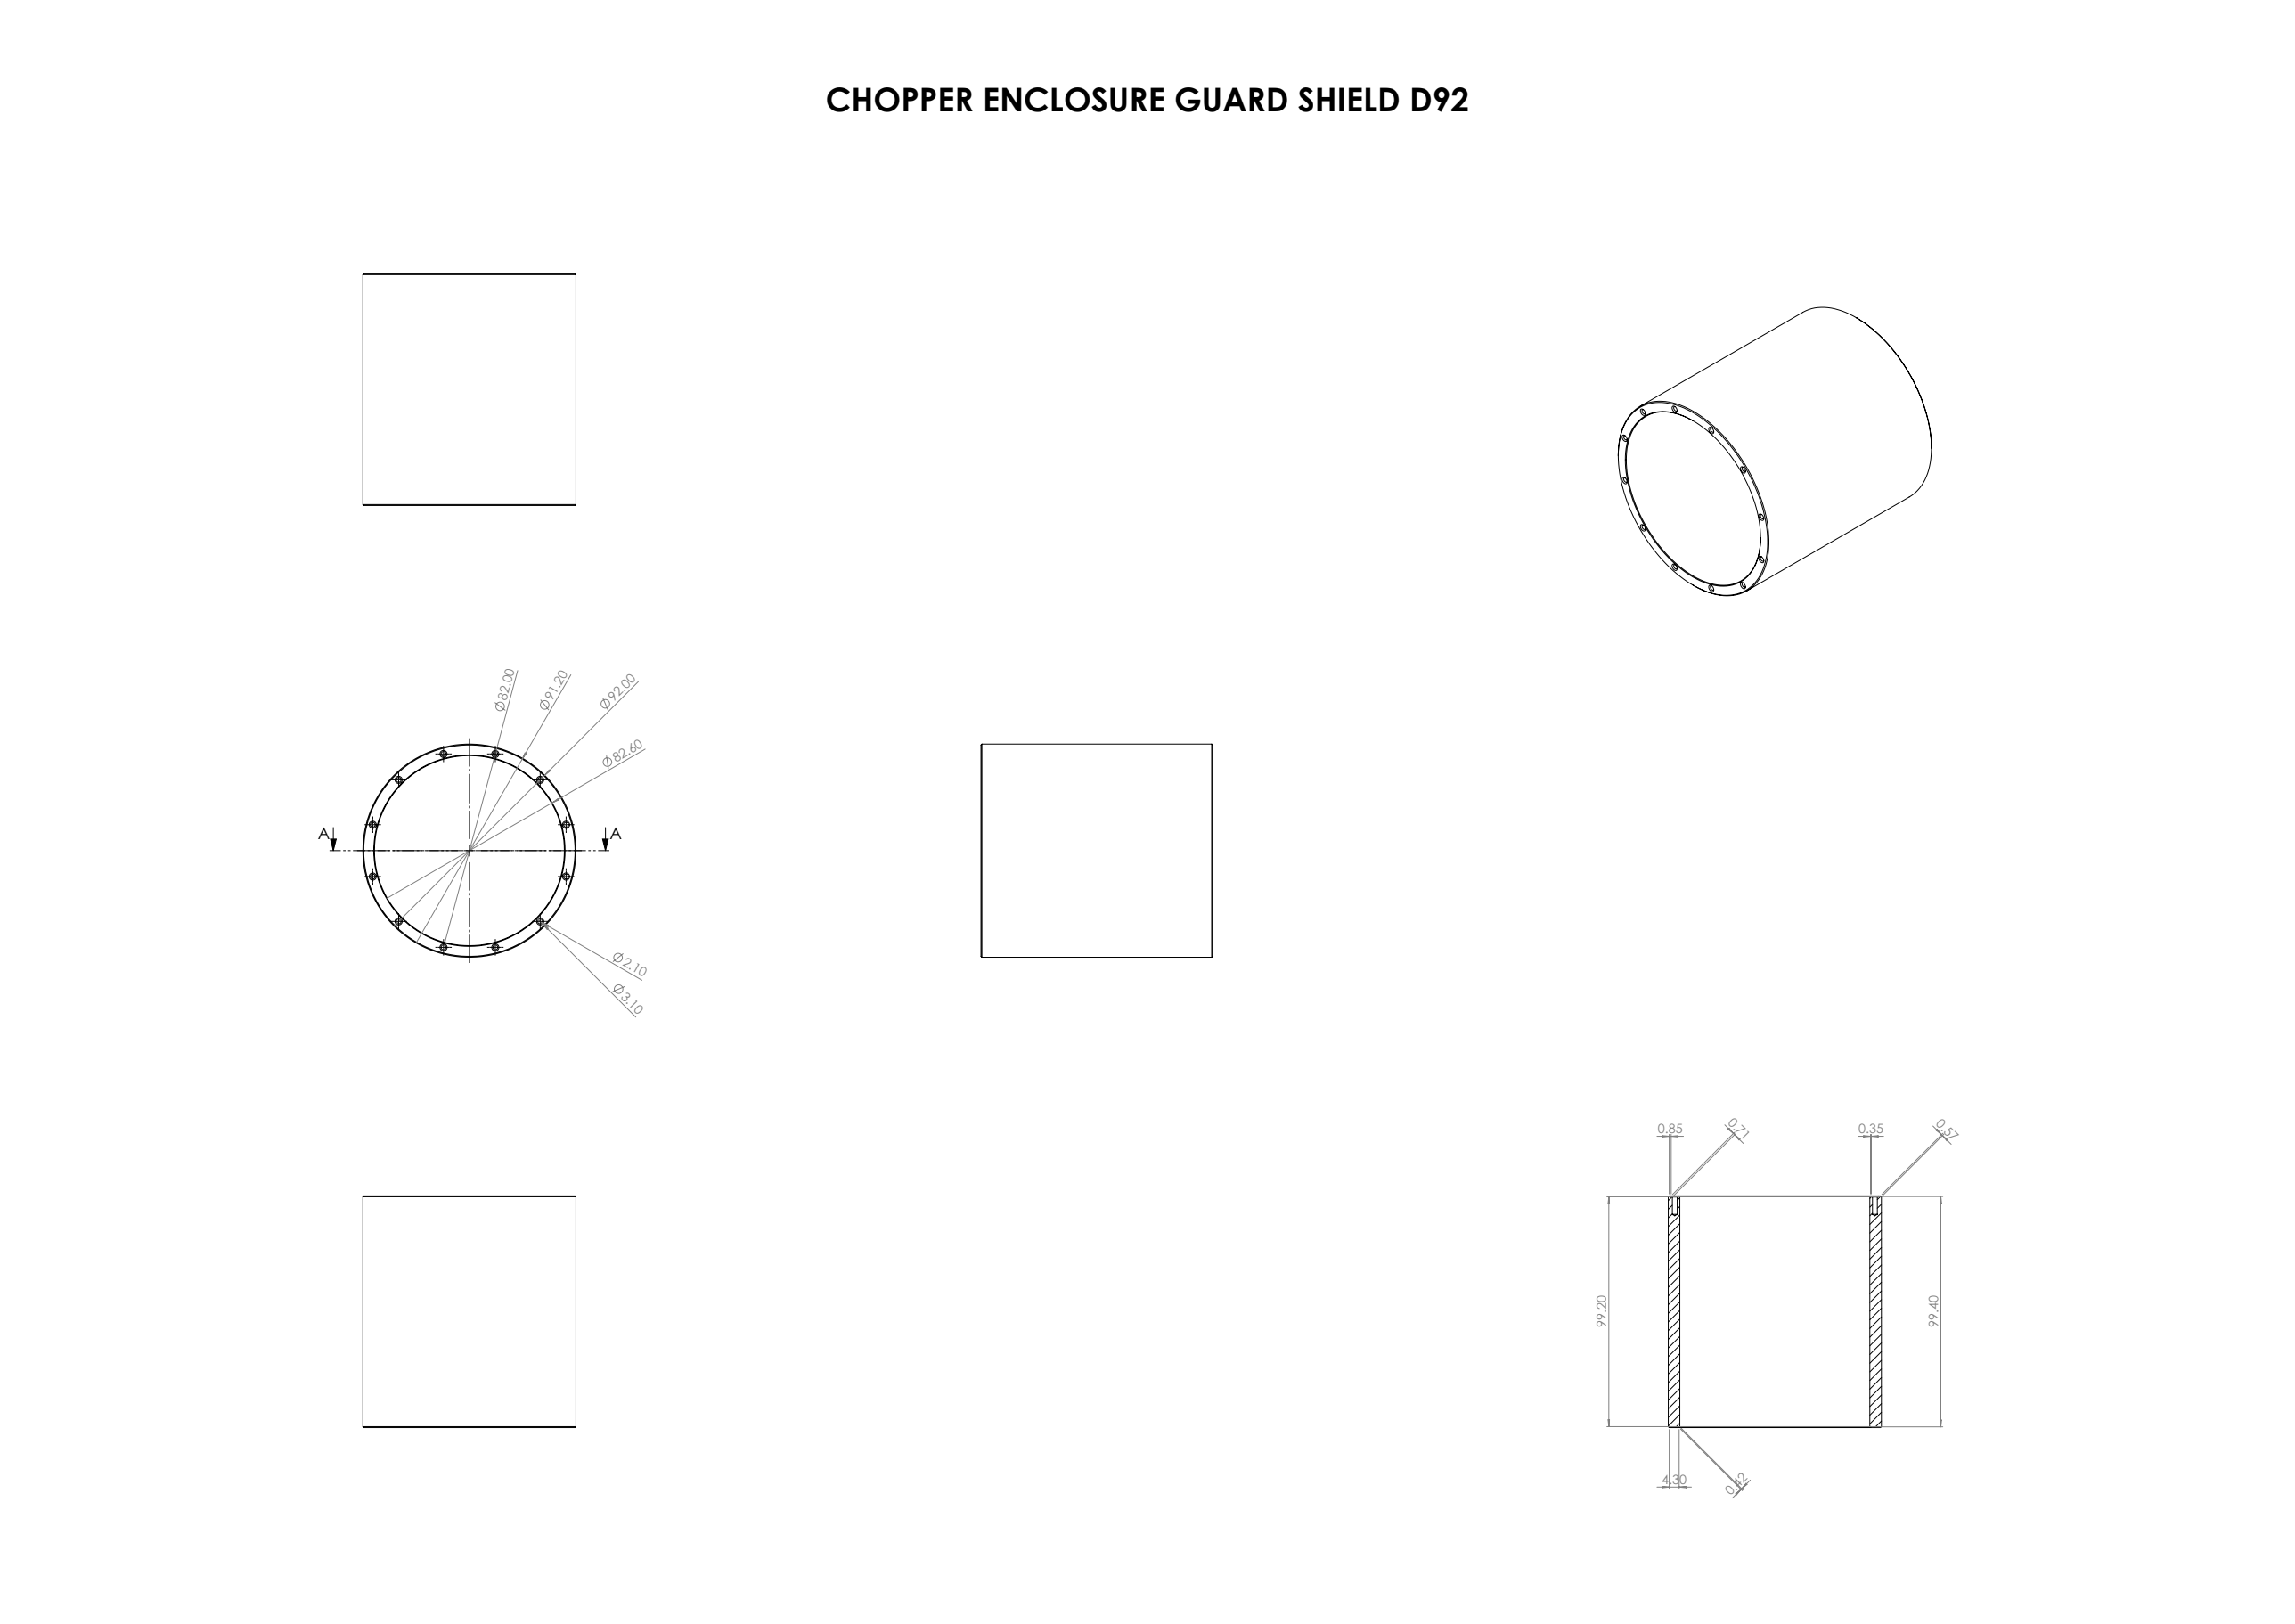
ISO-10303-21;
HEADER;
/* Generated by software containing ST-Developer
 * from STEP Tools, Inc. (www.steptools.com) 
 */

FILE_DESCRIPTION(
/* description */ (''),
/* implementation_level */ '2;1');

FILE_NAME(
/* name */ '02_Chopper_Enclosure_Guard_Shield_D92.step',
/* time_stamp */ '2026-10-19T23:00:43-07:00',
/* author */ (''),
/* organization */ (''),
/* preprocessor_version */ 'ST-DEVELOPER v20.2',
/* originating_system */ 'Autodesk Translation Framework v15.15.0.0',
/* authorisation */ '');

FILE_SCHEMA (('AUTOMOTIVE_DESIGN { 1 0 10303 214 3 1 1 }'));
ENDSEC;

DATA;
#10=MECHANICAL_DESIGN_GEOMETRIC_PRESENTATION_REPRESENTATION('',(#997),#55002);
#957=SHAPE_REPRESENTATION_RELATIONSHIP('SRR','None',#55105,#977);
#977=ADVANCED_BREP_SHAPE_REPRESENTATION('',(#1017),#54983);
#997=STYLED_ITEM('',(#55379),#1017);
#1017=MANIFOLD_SOLID_BREP('Enclosure Guard Shield',#24530);
#1062=FACE_BOUND('',#3929,.T.);
#1063=FACE_BOUND('',#3930,.T.);
#1064=FACE_BOUND('',#3931,.T.);
#1065=FACE_BOUND('',#3932,.T.);
#1066=FACE_BOUND('',#3933,.T.);
#1067=FACE_BOUND('',#3934,.T.);
#1068=FACE_BOUND('',#3935,.T.);
#1069=FACE_BOUND('',#3938,.T.);
#1070=FACE_BOUND('',#3939,.T.);
#1071=FACE_BOUND('',#3940,.T.);
#1072=FACE_BOUND('',#3941,.T.);
#1073=FACE_BOUND('',#3942,.T.);
#1074=FACE_BOUND('',#3943,.T.);
#1075=FACE_BOUND('',#3944,.T.);
#1076=FACE_BOUND('',#3945,.T.);
#1077=FACE_BOUND('',#3946,.T.);
#1078=FACE_BOUND('',#3947,.T.);
#1079=FACE_BOUND('',#3948,.T.);
#1080=FACE_BOUND('',#3949,.T.);
#1081=FACE_BOUND('',#3950,.T.);
#1287=PLANE('',#25045);
#1288=PLANE('',#25049);
#1972=CYLINDRICAL_SURFACE('',#24932,0.105);
#1973=CYLINDRICAL_SURFACE('',#24938,0.105);
#1974=CYLINDRICAL_SURFACE('',#24944,0.105);
#1975=CYLINDRICAL_SURFACE('',#24950,0.105);
#1976=CYLINDRICAL_SURFACE('',#24956,0.105);
#1977=CYLINDRICAL_SURFACE('',#24962,0.105);
#1978=CYLINDRICAL_SURFACE('',#24968,0.105);
#1979=CYLINDRICAL_SURFACE('',#24974,0.105);
#1980=CYLINDRICAL_SURFACE('',#24980,0.105);
#1981=CYLINDRICAL_SURFACE('',#24986,0.105);
#1982=CYLINDRICAL_SURFACE('',#24992,0.105);
#1983=CYLINDRICAL_SURFACE('',#24998,0.105);
#1984=CYLINDRICAL_SURFACE('',#25004,0.105);
#1985=CYLINDRICAL_SURFACE('',#25010,0.105);
#1986=CYLINDRICAL_SURFACE('',#25016,0.105);
#1987=CYLINDRICAL_SURFACE('',#25022,0.105);
#1988=CYLINDRICAL_SURFACE('',#25028,0.105);
#1989=CYLINDRICAL_SURFACE('',#25034,0.105);
#1990=CYLINDRICAL_SURFACE('',#25042,4.1);
#1991=CYLINDRICAL_SURFACE('',#25054,4.6);
#2482=FACE_OUTER_BOUND('',#3872,.T.);
#2483=FACE_OUTER_BOUND('',#3873,.T.);
#2484=FACE_OUTER_BOUND('',#3874,.T.);
#2485=FACE_OUTER_BOUND('',#3875,.T.);
#2486=FACE_OUTER_BOUND('',#3876,.T.);
#2487=FACE_OUTER_BOUND('',#3877,.T.);
#2488=FACE_OUTER_BOUND('',#3878,.T.);
#2489=FACE_OUTER_BOUND('',#3879,.T.);
#2490=FACE_OUTER_BOUND('',#3880,.T.);
#2491=FACE_OUTER_BOUND('',#3881,.T.);
#2492=FACE_OUTER_BOUND('',#3882,.T.);
#2493=FACE_OUTER_BOUND('',#3883,.T.);
#2494=FACE_OUTER_BOUND('',#3884,.T.);
#2495=FACE_OUTER_BOUND('',#3885,.T.);
#2496=FACE_OUTER_BOUND('',#3886,.T.);
#2497=FACE_OUTER_BOUND('',#3887,.T.);
#2498=FACE_OUTER_BOUND('',#3888,.T.);
#2499=FACE_OUTER_BOUND('',#3889,.T.);
#2500=FACE_OUTER_BOUND('',#3890,.T.);
#2501=FACE_OUTER_BOUND('',#3891,.T.);
#2502=FACE_OUTER_BOUND('',#3892,.T.);
#2503=FACE_OUTER_BOUND('',#3893,.T.);
#2504=FACE_OUTER_BOUND('',#3894,.T.);
#2505=FACE_OUTER_BOUND('',#3895,.T.);
#2506=FACE_OUTER_BOUND('',#3896,.T.);
#2507=FACE_OUTER_BOUND('',#3897,.T.);
#2508=FACE_OUTER_BOUND('',#3898,.T.);
#2509=FACE_OUTER_BOUND('',#3899,.T.);
#2510=FACE_OUTER_BOUND('',#3900,.T.);
#2511=FACE_OUTER_BOUND('',#3901,.T.);
#2512=FACE_OUTER_BOUND('',#3902,.T.);
#2513=FACE_OUTER_BOUND('',#3903,.T.);
#2514=FACE_OUTER_BOUND('',#3904,.T.);
#2515=FACE_OUTER_BOUND('',#3905,.T.);
#2516=FACE_OUTER_BOUND('',#3906,.T.);
#2517=FACE_OUTER_BOUND('',#3907,.T.);
#2518=FACE_OUTER_BOUND('',#3908,.T.);
#2519=FACE_OUTER_BOUND('',#3909,.T.);
#2520=FACE_OUTER_BOUND('',#3910,.T.);
#2521=FACE_OUTER_BOUND('',#3911,.T.);
#2522=FACE_OUTER_BOUND('',#3912,.T.);
#2523=FACE_OUTER_BOUND('',#3913,.T.);
#2524=FACE_OUTER_BOUND('',#3914,.T.);
#2525=FACE_OUTER_BOUND('',#3915,.T.);
#2526=FACE_OUTER_BOUND('',#3916,.T.);
#2527=FACE_OUTER_BOUND('',#3917,.T.);
#2528=FACE_OUTER_BOUND('',#3918,.T.);
#2529=FACE_OUTER_BOUND('',#3919,.T.);
#2530=FACE_OUTER_BOUND('',#3920,.T.);
#2531=FACE_OUTER_BOUND('',#3921,.T.);
#2532=FACE_OUTER_BOUND('',#3922,.T.);
#2533=FACE_OUTER_BOUND('',#3923,.T.);
#2534=FACE_OUTER_BOUND('',#3924,.T.);
#2535=FACE_OUTER_BOUND('',#3925,.T.);
#2536=FACE_OUTER_BOUND('',#3926,.T.);
#2537=FACE_OUTER_BOUND('',#3927,.T.);
#2538=FACE_OUTER_BOUND('',#3928,.T.);
#2539=FACE_OUTER_BOUND('',#3936,.T.);
#2540=FACE_OUTER_BOUND('',#3937,.T.);
#2541=FACE_OUTER_BOUND('',#3951,.T.);
#2542=FACE_OUTER_BOUND('',#3952,.T.);
#2543=FACE_OUTER_BOUND('',#3953,.T.);
#3872=EDGE_LOOP('',(#16178,#16179,#16180));
#3873=EDGE_LOOP('',(#16181,#16182,#16183,#16184));
#3874=EDGE_LOOP('',(#16185,#16186,#16187,#16188));
#3875=EDGE_LOOP('',(#16189,#16190,#16191));
#3876=EDGE_LOOP('',(#16192,#16193,#16194,#16195));
#3877=EDGE_LOOP('',(#16196,#16197,#16198,#16199));
#3878=EDGE_LOOP('',(#16200,#16201,#16202));
#3879=EDGE_LOOP('',(#16203,#16204,#16205,#16206));
#3880=EDGE_LOOP('',(#16207,#16208,#16209,#16210));
#3881=EDGE_LOOP('',(#16211,#16212,#16213));
#3882=EDGE_LOOP('',(#16214,#16215,#16216,#16217));
#3883=EDGE_LOOP('',(#16218,#16219,#16220,#16221));
#3884=EDGE_LOOP('',(#16222,#16223,#16224));
#3885=EDGE_LOOP('',(#16225,#16226,#16227,#16228));
#3886=EDGE_LOOP('',(#16229,#16230,#16231,#16232));
#3887=EDGE_LOOP('',(#16233,#16234,#16235));
#3888=EDGE_LOOP('',(#16236,#16237,#16238,#16239));
#3889=EDGE_LOOP('',(#16240,#16241,#16242,#16243));
#3890=EDGE_LOOP('',(#16244,#16245,#16246));
#3891=EDGE_LOOP('',(#16247,#16248,#16249,#16250));
#3892=EDGE_LOOP('',(#16251,#16252,#16253,#16254));
#3893=EDGE_LOOP('',(#16255,#16256,#16257));
#3894=EDGE_LOOP('',(#16258,#16259,#16260,#16261));
#3895=EDGE_LOOP('',(#16262,#16263,#16264,#16265));
#3896=EDGE_LOOP('',(#16266,#16267,#16268));
#3897=EDGE_LOOP('',(#16269,#16270,#16271,#16272));
#3898=EDGE_LOOP('',(#16273,#16274,#16275,#16276));
#3899=EDGE_LOOP('',(#16277,#16278,#16279));
#3900=EDGE_LOOP('',(#16280,#16281,#16282,#16283));
#3901=EDGE_LOOP('',(#16284,#16285,#16286,#16287));
#3902=EDGE_LOOP('',(#16288,#16289,#16290));
#3903=EDGE_LOOP('',(#16291,#16292,#16293,#16294));
#3904=EDGE_LOOP('',(#16295,#16296,#16297,#16298));
#3905=EDGE_LOOP('',(#16299,#16300,#16301));
#3906=EDGE_LOOP('',(#16302,#16303,#16304,#16305));
#3907=EDGE_LOOP('',(#16306,#16307,#16308,#16309));
#3908=EDGE_LOOP('',(#16310,#16311,#16312));
#3909=EDGE_LOOP('',(#16313,#16314,#16315,#16316));
#3910=EDGE_LOOP('',(#16317,#16318,#16319,#16320));
#3911=EDGE_LOOP('',(#16321,#16322,#16323));
#3912=EDGE_LOOP('',(#16324,#16325,#16326,#16327));
#3913=EDGE_LOOP('',(#16328,#16329,#16330,#16331));
#3914=EDGE_LOOP('',(#16332,#16333,#16334));
#3915=EDGE_LOOP('',(#16335,#16336,#16337,#16338));
#3916=EDGE_LOOP('',(#16339,#16340,#16341,#16342));
#3917=EDGE_LOOP('',(#16343,#16344,#16345));
#3918=EDGE_LOOP('',(#16346,#16347,#16348,#16349));
#3919=EDGE_LOOP('',(#16350,#16351,#16352,#16353));
#3920=EDGE_LOOP('',(#16354,#16355,#16356));
#3921=EDGE_LOOP('',(#16357,#16358,#16359,#16360));
#3922=EDGE_LOOP('',(#16361,#16362,#16363,#16364));
#3923=EDGE_LOOP('',(#16365,#16366,#16367));
#3924=EDGE_LOOP('',(#16368,#16369,#16370,#16371));
#3925=EDGE_LOOP('',(#16372,#16373,#16374,#16375));
#3926=EDGE_LOOP('',(#16376,#16377,#16378,#16379,#16380));
#3927=EDGE_LOOP('',(#16381,#16382,#16383,#16384,#16385,#16386));
#3928=EDGE_LOOP('',(#16387));
#3929=EDGE_LOOP('',(#16388));
#3930=EDGE_LOOP('',(#16389));
#3931=EDGE_LOOP('',(#16390));
#3932=EDGE_LOOP('',(#16391));
#3933=EDGE_LOOP('',(#16392));
#3934=EDGE_LOOP('',(#16393));
#3935=EDGE_LOOP('',(#16394));
#3936=EDGE_LOOP('',(#16395,#16396,#16397,#16398,#16399));
#3937=EDGE_LOOP('',(#16400));
#3938=EDGE_LOOP('',(#16401));
#3939=EDGE_LOOP('',(#16402));
#3940=EDGE_LOOP('',(#16403));
#3941=EDGE_LOOP('',(#16404));
#3942=EDGE_LOOP('',(#16405));
#3943=EDGE_LOOP('',(#16406));
#3944=EDGE_LOOP('',(#16407));
#3945=EDGE_LOOP('',(#16408));
#3946=EDGE_LOOP('',(#16409));
#3947=EDGE_LOOP('',(#16410));
#3948=EDGE_LOOP('',(#16411));
#3949=EDGE_LOOP('',(#16412));
#3950=EDGE_LOOP('',(#16413));
#3951=EDGE_LOOP('',(#16414,#16415,#16416,#16417,#16418));
#3952=EDGE_LOOP('',(#16419,#16420,#16421,#16422,#16423,#16424));
#3953=EDGE_LOOP('',(#16425,#16426,#16427,#16428,#16429));
#5439=LINE('',#34181,#7260);
#5440=LINE('',#34185,#7261);
#5441=LINE('',#34189,#7262);
#5442=LINE('',#34194,#7263);
#5443=LINE('',#34198,#7264);
#5444=LINE('',#34202,#7265);
#5445=LINE('',#34207,#7266);
#5446=LINE('',#34211,#7267);
#5447=LINE('',#34215,#7268);
#5448=LINE('',#34220,#7269);
#5449=LINE('',#34224,#7270);
#5450=LINE('',#34228,#7271);
#5451=LINE('',#34233,#7272);
#5452=LINE('',#34237,#7273);
#5453=LINE('',#34241,#7274);
#5454=LINE('',#34246,#7275);
#5455=LINE('',#34250,#7276);
#5456=LINE('',#34254,#7277);
#5457=LINE('',#34259,#7278);
#5458=LINE('',#34263,#7279);
#5459=LINE('',#34267,#7280);
#5460=LINE('',#34272,#7281);
#5461=LINE('',#34276,#7282);
#5462=LINE('',#34280,#7283);
#5463=LINE('',#34285,#7284);
#5464=LINE('',#34289,#7285);
#5465=LINE('',#34293,#7286);
#5466=LINE('',#34298,#7287);
#5467=LINE('',#34302,#7288);
#5468=LINE('',#34306,#7289);
#5469=LINE('',#34311,#7290);
#5470=LINE('',#34315,#7291);
#5471=LINE('',#34319,#7292);
#5472=LINE('',#34324,#7293);
#5473=LINE('',#34328,#7294);
#5474=LINE('',#34332,#7295);
#5475=LINE('',#34337,#7296);
#5476=LINE('',#34341,#7297);
#5477=LINE('',#34345,#7298);
#5478=LINE('',#34350,#7299);
#5479=LINE('',#34354,#7300);
#5480=LINE('',#34358,#7301);
#5481=LINE('',#34363,#7302);
#5482=LINE('',#34367,#7303);
#5483=LINE('',#34371,#7304);
#5484=LINE('',#34376,#7305);
#5485=LINE('',#34380,#7306);
#5486=LINE('',#34384,#7307);
#5487=LINE('',#34389,#7308);
#5488=LINE('',#34393,#7309);
#5489=LINE('',#34397,#7310);
#5490=LINE('',#34402,#7311);
#5491=LINE('',#34406,#7312);
#5492=LINE('',#34410,#7313);
#5493=LINE('',#34416,#7314);
#5494=LINE('',#34425,#7315);
#5495=LINE('',#34431,#7316);
#5496=LINE('',#34438,#7317);
#5497=LINE('',#34444,#7318);
#5498=LINE('',#34449,#7319);
#7260=VECTOR('',#27577,0.0524999999999998);
#7261=VECTOR('',#27582,0.105);
#7262=VECTOR('',#27587,0.155);
#7263=VECTOR('',#27592,0.0525000000000002);
#7264=VECTOR('',#27597,0.105);
#7265=VECTOR('',#27602,0.155);
#7266=VECTOR('',#27607,0.0525000000000002);
#7267=VECTOR('',#27612,0.105);
#7268=VECTOR('',#27617,0.154999999999999);
#7269=VECTOR('',#27622,0.0525000000000002);
#7270=VECTOR('',#27627,0.105);
#7271=VECTOR('',#27632,0.155);
#7272=VECTOR('',#27637,0.0524999999999998);
#7273=VECTOR('',#27642,0.105);
#7274=VECTOR('',#27647,0.155);
#7275=VECTOR('',#27652,0.0525000000000002);
#7276=VECTOR('',#27657,0.105);
#7277=VECTOR('',#27662,0.154999999999999);
#7278=VECTOR('',#27667,0.0525000000000002);
#7279=VECTOR('',#27672,0.105);
#7280=VECTOR('',#27677,0.154999999999999);
#7281=VECTOR('',#27682,0.0524999999999998);
#7282=VECTOR('',#27687,0.105);
#7283=VECTOR('',#27692,0.155);
#7284=VECTOR('',#27697,0.0525);
#7285=VECTOR('',#27702,0.105);
#7286=VECTOR('',#27707,0.155);
#7287=VECTOR('',#27712,0.0525);
#7288=VECTOR('',#27717,0.105);
#7289=VECTOR('',#27722,0.155);
#7290=VECTOR('',#27727,0.0525000000000002);
#7291=VECTOR('',#27732,0.105);
#7292=VECTOR('',#27737,0.155);
#7293=VECTOR('',#27742,0.0525000000000002);
#7294=VECTOR('',#27747,0.105);
#7295=VECTOR('',#27752,0.155);
#7296=VECTOR('',#27757,0.0524999999999993);
#7297=VECTOR('',#27762,0.105);
#7298=VECTOR('',#27767,0.155);
#7299=VECTOR('',#27772,0.0525000000000002);
#7300=VECTOR('',#27777,0.105);
#7301=VECTOR('',#27782,0.155);
#7302=VECTOR('',#27787,0.0525);
#7303=VECTOR('',#27792,0.105);
#7304=VECTOR('',#27797,0.155);
#7305=VECTOR('',#27802,0.0525);
#7306=VECTOR('',#27807,0.105);
#7307=VECTOR('',#27812,0.155);
#7308=VECTOR('',#27817,0.0524999999999998);
#7309=VECTOR('',#27822,0.105);
#7310=VECTOR('',#27827,0.155);
#7311=VECTOR('',#27832,0.0525000000000002);
#7312=VECTOR('',#27837,0.105);
#7313=VECTOR('',#27842,0.154999999999999);
#7314=VECTOR('',#27849,4.115);
#7315=VECTOR('',#27860,4.1);
#7316=VECTOR('',#27867,4.115);
#7317=VECTOR('',#27876,4.58);
#7318=VECTOR('',#27883,4.6);
#7319=VECTOR('',#27890,4.58);
#9109=CIRCLE('',#24931,0.105);
#9110=CIRCLE('',#24933,0.105);
#9111=CIRCLE('',#24935,0.155);
#9112=CIRCLE('',#24937,0.105);
#9113=CIRCLE('',#24939,0.105);
#9114=CIRCLE('',#24941,0.155);
#9115=CIRCLE('',#24943,0.105);
#9116=CIRCLE('',#24945,0.105);
#9117=CIRCLE('',#24947,0.154999999999999);
#9118=CIRCLE('',#24949,0.105);
#9119=CIRCLE('',#24951,0.105);
#9120=CIRCLE('',#24953,0.155);
#9121=CIRCLE('',#24955,0.105);
#9122=CIRCLE('',#24957,0.105);
#9123=CIRCLE('',#24959,0.155);
#9124=CIRCLE('',#24961,0.105);
#9125=CIRCLE('',#24963,0.105);
#9126=CIRCLE('',#24965,0.154999999999999);
#9127=CIRCLE('',#24967,0.105);
#9128=CIRCLE('',#24969,0.105);
#9129=CIRCLE('',#24971,0.154999999999999);
#9130=CIRCLE('',#24973,0.105);
#9131=CIRCLE('',#24975,0.105);
#9132=CIRCLE('',#24977,0.155);
#9133=CIRCLE('',#24979,0.105);
#9134=CIRCLE('',#24981,0.105);
#9135=CIRCLE('',#24983,0.155);
#9136=CIRCLE('',#24985,0.105);
#9137=CIRCLE('',#24987,0.105);
#9138=CIRCLE('',#24989,0.155);
#9139=CIRCLE('',#24991,0.105);
#9140=CIRCLE('',#24993,0.105);
#9141=CIRCLE('',#24995,0.155);
#9142=CIRCLE('',#24997,0.105);
#9143=CIRCLE('',#24999,0.105);
#9144=CIRCLE('',#25001,0.155);
#9145=CIRCLE('',#25003,0.105);
#9146=CIRCLE('',#25005,0.105);
#9147=CIRCLE('',#25007,0.155);
#9148=CIRCLE('',#25009,0.105);
#9149=CIRCLE('',#25011,0.105);
#9150=CIRCLE('',#25013,0.155);
#9151=CIRCLE('',#25015,0.105);
#9152=CIRCLE('',#25017,0.105);
#9153=CIRCLE('',#25019,0.155);
#9154=CIRCLE('',#25021,0.105);
#9155=CIRCLE('',#25023,0.105);
#9156=CIRCLE('',#25025,0.155);
#9157=CIRCLE('',#25027,0.105);
#9158=CIRCLE('',#25029,0.105);
#9159=CIRCLE('',#25031,0.155);
#9160=CIRCLE('',#25033,0.105);
#9161=CIRCLE('',#25035,0.105);
#9162=CIRCLE('',#25037,0.154999999999999);
#9163=CIRCLE('',#25039,4.13);
#9164=CIRCLE('',#25040,4.1);
#9165=CIRCLE('',#25041,4.1);
#9166=CIRCLE('',#25043,4.1);
#9167=CIRCLE('',#25044,4.1);
#9168=CIRCLE('',#25046,4.56);
#9169=CIRCLE('',#25048,4.13);
#9170=CIRCLE('',#25050,4.56);
#9171=CIRCLE('',#25052,4.6);
#9172=CIRCLE('',#25053,4.6);
#9173=CIRCLE('',#25055,4.6);
#9174=CIRCLE('',#25056,4.6);
#10116=VERTEX_POINT('',#34179);
#10117=VERTEX_POINT('',#34180);
#10118=VERTEX_POINT('',#34184);
#10119=VERTEX_POINT('',#34188);
#10120=VERTEX_POINT('',#34192);
#10121=VERTEX_POINT('',#34193);
#10122=VERTEX_POINT('',#34197);
#10123=VERTEX_POINT('',#34201);
#10124=VERTEX_POINT('',#34205);
#10125=VERTEX_POINT('',#34206);
#10126=VERTEX_POINT('',#34210);
#10127=VERTEX_POINT('',#34214);
#10128=VERTEX_POINT('',#34218);
#10129=VERTEX_POINT('',#34219);
#10130=VERTEX_POINT('',#34223);
#10131=VERTEX_POINT('',#34227);
#10132=VERTEX_POINT('',#34231);
#10133=VERTEX_POINT('',#34232);
#10134=VERTEX_POINT('',#34236);
#10135=VERTEX_POINT('',#34240);
#10136=VERTEX_POINT('',#34244);
#10137=VERTEX_POINT('',#34245);
#10138=VERTEX_POINT('',#34249);
#10139=VERTEX_POINT('',#34253);
#10140=VERTEX_POINT('',#34257);
#10141=VERTEX_POINT('',#34258);
#10142=VERTEX_POINT('',#34262);
#10143=VERTEX_POINT('',#34266);
#10144=VERTEX_POINT('',#34270);
#10145=VERTEX_POINT('',#34271);
#10146=VERTEX_POINT('',#34275);
#10147=VERTEX_POINT('',#34279);
#10148=VERTEX_POINT('',#34283);
#10149=VERTEX_POINT('',#34284);
#10150=VERTEX_POINT('',#34288);
#10151=VERTEX_POINT('',#34292);
#10152=VERTEX_POINT('',#34296);
#10153=VERTEX_POINT('',#34297);
#10154=VERTEX_POINT('',#34301);
#10155=VERTEX_POINT('',#34305);
#10156=VERTEX_POINT('',#34309);
#10157=VERTEX_POINT('',#34310);
#10158=VERTEX_POINT('',#34314);
#10159=VERTEX_POINT('',#34318);
#10160=VERTEX_POINT('',#34322);
#10161=VERTEX_POINT('',#34323);
#10162=VERTEX_POINT('',#34327);
#10163=VERTEX_POINT('',#34331);
#10164=VERTEX_POINT('',#34335);
#10165=VERTEX_POINT('',#34336);
#10166=VERTEX_POINT('',#34340);
#10167=VERTEX_POINT('',#34344);
#10168=VERTEX_POINT('',#34348);
#10169=VERTEX_POINT('',#34349);
#10170=VERTEX_POINT('',#34353);
#10171=VERTEX_POINT('',#34357);
#10172=VERTEX_POINT('',#34361);
#10173=VERTEX_POINT('',#34362);
#10174=VERTEX_POINT('',#34366);
#10175=VERTEX_POINT('',#34370);
#10176=VERTEX_POINT('',#34374);
#10177=VERTEX_POINT('',#34375);
#10178=VERTEX_POINT('',#34379);
#10179=VERTEX_POINT('',#34383);
#10180=VERTEX_POINT('',#34387);
#10181=VERTEX_POINT('',#34388);
#10182=VERTEX_POINT('',#34392);
#10183=VERTEX_POINT('',#34396);
#10184=VERTEX_POINT('',#34400);
#10185=VERTEX_POINT('',#34401);
#10186=VERTEX_POINT('',#34405);
#10187=VERTEX_POINT('',#34409);
#10188=VERTEX_POINT('',#34413);
#10189=VERTEX_POINT('',#34415);
#10190=VERTEX_POINT('',#34417);
#10191=VERTEX_POINT('',#34421);
#10192=VERTEX_POINT('',#34422);
#10193=VERTEX_POINT('',#34427);
#10194=VERTEX_POINT('',#34430);
#10195=VERTEX_POINT('',#34434);
#10196=VERTEX_POINT('',#34437);
#10197=VERTEX_POINT('',#34439);
#10198=VERTEX_POINT('',#34443);
#10199=VERTEX_POINT('',#34445);
#12497=EDGE_CURVE('',#10116,#10117,#5439,.T.);
#12498=EDGE_CURVE('',#10117,#10117,#9109,.T.);
#12499=EDGE_CURVE('',#10117,#10118,#5440,.T.);
#12500=EDGE_CURVE('',#10118,#10118,#9110,.T.);
#12501=EDGE_CURVE('',#10118,#10119,#5441,.T.);
#12502=EDGE_CURVE('',#10119,#10119,#9111,.T.);
#12503=EDGE_CURVE('',#10120,#10121,#5442,.T.);
#12504=EDGE_CURVE('',#10121,#10121,#9112,.T.);
#12505=EDGE_CURVE('',#10121,#10122,#5443,.T.);
#12506=EDGE_CURVE('',#10122,#10122,#9113,.T.);
#12507=EDGE_CURVE('',#10122,#10123,#5444,.T.);
#12508=EDGE_CURVE('',#10123,#10123,#9114,.T.);
#12509=EDGE_CURVE('',#10124,#10125,#5445,.T.);
#12510=EDGE_CURVE('',#10125,#10125,#9115,.T.);
#12511=EDGE_CURVE('',#10125,#10126,#5446,.T.);
#12512=EDGE_CURVE('',#10126,#10126,#9116,.T.);
#12513=EDGE_CURVE('',#10126,#10127,#5447,.T.);
#12514=EDGE_CURVE('',#10127,#10127,#9117,.T.);
#12515=EDGE_CURVE('',#10128,#10129,#5448,.T.);
#12516=EDGE_CURVE('',#10129,#10129,#9118,.T.);
#12517=EDGE_CURVE('',#10129,#10130,#5449,.T.);
#12518=EDGE_CURVE('',#10130,#10130,#9119,.T.);
#12519=EDGE_CURVE('',#10130,#10131,#5450,.T.);
#12520=EDGE_CURVE('',#10131,#10131,#9120,.T.);
#12521=EDGE_CURVE('',#10132,#10133,#5451,.T.);
#12522=EDGE_CURVE('',#10133,#10133,#9121,.T.);
#12523=EDGE_CURVE('',#10133,#10134,#5452,.T.);
#12524=EDGE_CURVE('',#10134,#10134,#9122,.T.);
#12525=EDGE_CURVE('',#10134,#10135,#5453,.T.);
#12526=EDGE_CURVE('',#10135,#10135,#9123,.T.);
#12527=EDGE_CURVE('',#10136,#10137,#5454,.T.);
#12528=EDGE_CURVE('',#10137,#10137,#9124,.T.);
#12529=EDGE_CURVE('',#10137,#10138,#5455,.T.);
#12530=EDGE_CURVE('',#10138,#10138,#9125,.T.);
#12531=EDGE_CURVE('',#10138,#10139,#5456,.T.);
#12532=EDGE_CURVE('',#10139,#10139,#9126,.T.);
#12533=EDGE_CURVE('',#10140,#10141,#5457,.T.);
#12534=EDGE_CURVE('',#10141,#10141,#9127,.T.);
#12535=EDGE_CURVE('',#10141,#10142,#5458,.T.);
#12536=EDGE_CURVE('',#10142,#10142,#9128,.T.);
#12537=EDGE_CURVE('',#10142,#10143,#5459,.T.);
#12538=EDGE_CURVE('',#10143,#10143,#9129,.T.);
#12539=EDGE_CURVE('',#10144,#10145,#5460,.T.);
#12540=EDGE_CURVE('',#10145,#10145,#9130,.T.);
#12541=EDGE_CURVE('',#10145,#10146,#5461,.T.);
#12542=EDGE_CURVE('',#10146,#10146,#9131,.T.);
#12543=EDGE_CURVE('',#10146,#10147,#5462,.T.);
#12544=EDGE_CURVE('',#10147,#10147,#9132,.T.);
#12545=EDGE_CURVE('',#10148,#10149,#5463,.T.);
#12546=EDGE_CURVE('',#10149,#10149,#9133,.T.);
#12547=EDGE_CURVE('',#10149,#10150,#5464,.T.);
#12548=EDGE_CURVE('',#10150,#10150,#9134,.T.);
#12549=EDGE_CURVE('',#10150,#10151,#5465,.T.);
#12550=EDGE_CURVE('',#10151,#10151,#9135,.T.);
#12551=EDGE_CURVE('',#10152,#10153,#5466,.T.);
#12552=EDGE_CURVE('',#10153,#10153,#9136,.T.);
#12553=EDGE_CURVE('',#10153,#10154,#5467,.T.);
#12554=EDGE_CURVE('',#10154,#10154,#9137,.T.);
#12555=EDGE_CURVE('',#10154,#10155,#5468,.T.);
#12556=EDGE_CURVE('',#10155,#10155,#9138,.T.);
#12557=EDGE_CURVE('',#10156,#10157,#5469,.T.);
#12558=EDGE_CURVE('',#10157,#10157,#9139,.T.);
#12559=EDGE_CURVE('',#10157,#10158,#5470,.T.);
#12560=EDGE_CURVE('',#10158,#10158,#9140,.T.);
#12561=EDGE_CURVE('',#10158,#10159,#5471,.T.);
#12562=EDGE_CURVE('',#10159,#10159,#9141,.T.);
#12563=EDGE_CURVE('',#10160,#10161,#5472,.T.);
#12564=EDGE_CURVE('',#10161,#10161,#9142,.T.);
#12565=EDGE_CURVE('',#10161,#10162,#5473,.T.);
#12566=EDGE_CURVE('',#10162,#10162,#9143,.T.);
#12567=EDGE_CURVE('',#10162,#10163,#5474,.T.);
#12568=EDGE_CURVE('',#10163,#10163,#9144,.T.);
#12569=EDGE_CURVE('',#10164,#10165,#5475,.T.);
#12570=EDGE_CURVE('',#10165,#10165,#9145,.T.);
#12571=EDGE_CURVE('',#10165,#10166,#5476,.T.);
#12572=EDGE_CURVE('',#10166,#10166,#9146,.T.);
#12573=EDGE_CURVE('',#10166,#10167,#5477,.T.);
#12574=EDGE_CURVE('',#10167,#10167,#9147,.T.);
#12575=EDGE_CURVE('',#10168,#10169,#5478,.T.);
#12576=EDGE_CURVE('',#10169,#10169,#9148,.T.);
#12577=EDGE_CURVE('',#10169,#10170,#5479,.T.);
#12578=EDGE_CURVE('',#10170,#10170,#9149,.T.);
#12579=EDGE_CURVE('',#10170,#10171,#5480,.T.);
#12580=EDGE_CURVE('',#10171,#10171,#9150,.T.);
#12581=EDGE_CURVE('',#10172,#10173,#5481,.T.);
#12582=EDGE_CURVE('',#10173,#10173,#9151,.T.);
#12583=EDGE_CURVE('',#10173,#10174,#5482,.T.);
#12584=EDGE_CURVE('',#10174,#10174,#9152,.T.);
#12585=EDGE_CURVE('',#10174,#10175,#5483,.T.);
#12586=EDGE_CURVE('',#10175,#10175,#9153,.T.);
#12587=EDGE_CURVE('',#10176,#10177,#5484,.T.);
#12588=EDGE_CURVE('',#10177,#10177,#9154,.T.);
#12589=EDGE_CURVE('',#10177,#10178,#5485,.T.);
#12590=EDGE_CURVE('',#10178,#10178,#9155,.T.);
#12591=EDGE_CURVE('',#10178,#10179,#5486,.T.);
#12592=EDGE_CURVE('',#10179,#10179,#9156,.T.);
#12593=EDGE_CURVE('',#10180,#10181,#5487,.T.);
#12594=EDGE_CURVE('',#10181,#10181,#9157,.T.);
#12595=EDGE_CURVE('',#10181,#10182,#5488,.T.);
#12596=EDGE_CURVE('',#10182,#10182,#9158,.T.);
#12597=EDGE_CURVE('',#10182,#10183,#5489,.T.);
#12598=EDGE_CURVE('',#10183,#10183,#9159,.T.);
#12599=EDGE_CURVE('',#10184,#10185,#5490,.T.);
#12600=EDGE_CURVE('',#10185,#10185,#9160,.T.);
#12601=EDGE_CURVE('',#10185,#10186,#5491,.T.);
#12602=EDGE_CURVE('',#10186,#10186,#9161,.T.);
#12603=EDGE_CURVE('',#10186,#10187,#5492,.T.);
#12604=EDGE_CURVE('',#10187,#10187,#9162,.T.);
#12605=EDGE_CURVE('',#10188,#10188,#9163,.T.);
#12606=EDGE_CURVE('',#10188,#10189,#5493,.T.);
#12607=EDGE_CURVE('',#10189,#10190,#9164,.T.);
#12608=EDGE_CURVE('',#10190,#10189,#9165,.T.);
#12609=EDGE_CURVE('',#10191,#10192,#9166,.T.);
#12610=EDGE_CURVE('',#10192,#10191,#9167,.T.);
#12611=EDGE_CURVE('',#10192,#10190,#5494,.T.);
#12612=EDGE_CURVE('',#10193,#10193,#9168,.T.);
#12613=EDGE_CURVE('',#10191,#10194,#5495,.T.);
#12614=EDGE_CURVE('',#10194,#10194,#9169,.T.);
#12615=EDGE_CURVE('',#10195,#10195,#9170,.T.);
#12616=EDGE_CURVE('',#10195,#10196,#5496,.T.);
#12617=EDGE_CURVE('',#10196,#10197,#9171,.T.);
#12618=EDGE_CURVE('',#10197,#10196,#9172,.T.);
#12619=EDGE_CURVE('',#10197,#10198,#5497,.T.);
#12620=EDGE_CURVE('',#10199,#10198,#9173,.T.);
#12621=EDGE_CURVE('',#10198,#10199,#9174,.T.);
#12622=EDGE_CURVE('',#10199,#10193,#5498,.T.);
#16178=ORIENTED_EDGE('',*,*,#12497,.T.);
#16179=ORIENTED_EDGE('',*,*,#12498,.T.);
#16180=ORIENTED_EDGE('',*,*,#12497,.F.);
#16181=ORIENTED_EDGE('',*,*,#12498,.F.);
#16182=ORIENTED_EDGE('',*,*,#12499,.T.);
#16183=ORIENTED_EDGE('',*,*,#12500,.T.);
#16184=ORIENTED_EDGE('',*,*,#12499,.F.);
#16185=ORIENTED_EDGE('',*,*,#12500,.F.);
#16186=ORIENTED_EDGE('',*,*,#12501,.T.);
#16187=ORIENTED_EDGE('',*,*,#12502,.F.);
#16188=ORIENTED_EDGE('',*,*,#12501,.F.);
#16189=ORIENTED_EDGE('',*,*,#12503,.T.);
#16190=ORIENTED_EDGE('',*,*,#12504,.T.);
#16191=ORIENTED_EDGE('',*,*,#12503,.F.);
#16192=ORIENTED_EDGE('',*,*,#12504,.F.);
#16193=ORIENTED_EDGE('',*,*,#12505,.T.);
#16194=ORIENTED_EDGE('',*,*,#12506,.T.);
#16195=ORIENTED_EDGE('',*,*,#12505,.F.);
#16196=ORIENTED_EDGE('',*,*,#12506,.F.);
#16197=ORIENTED_EDGE('',*,*,#12507,.T.);
#16198=ORIENTED_EDGE('',*,*,#12508,.F.);
#16199=ORIENTED_EDGE('',*,*,#12507,.F.);
#16200=ORIENTED_EDGE('',*,*,#12509,.T.);
#16201=ORIENTED_EDGE('',*,*,#12510,.T.);
#16202=ORIENTED_EDGE('',*,*,#12509,.F.);
#16203=ORIENTED_EDGE('',*,*,#12510,.F.);
#16204=ORIENTED_EDGE('',*,*,#12511,.T.);
#16205=ORIENTED_EDGE('',*,*,#12512,.T.);
#16206=ORIENTED_EDGE('',*,*,#12511,.F.);
#16207=ORIENTED_EDGE('',*,*,#12512,.F.);
#16208=ORIENTED_EDGE('',*,*,#12513,.T.);
#16209=ORIENTED_EDGE('',*,*,#12514,.F.);
#16210=ORIENTED_EDGE('',*,*,#12513,.F.);
#16211=ORIENTED_EDGE('',*,*,#12515,.T.);
#16212=ORIENTED_EDGE('',*,*,#12516,.T.);
#16213=ORIENTED_EDGE('',*,*,#12515,.F.);
#16214=ORIENTED_EDGE('',*,*,#12516,.F.);
#16215=ORIENTED_EDGE('',*,*,#12517,.T.);
#16216=ORIENTED_EDGE('',*,*,#12518,.T.);
#16217=ORIENTED_EDGE('',*,*,#12517,.F.);
#16218=ORIENTED_EDGE('',*,*,#12518,.F.);
#16219=ORIENTED_EDGE('',*,*,#12519,.T.);
#16220=ORIENTED_EDGE('',*,*,#12520,.F.);
#16221=ORIENTED_EDGE('',*,*,#12519,.F.);
#16222=ORIENTED_EDGE('',*,*,#12521,.T.);
#16223=ORIENTED_EDGE('',*,*,#12522,.T.);
#16224=ORIENTED_EDGE('',*,*,#12521,.F.);
#16225=ORIENTED_EDGE('',*,*,#12522,.F.);
#16226=ORIENTED_EDGE('',*,*,#12523,.T.);
#16227=ORIENTED_EDGE('',*,*,#12524,.T.);
#16228=ORIENTED_EDGE('',*,*,#12523,.F.);
#16229=ORIENTED_EDGE('',*,*,#12524,.F.);
#16230=ORIENTED_EDGE('',*,*,#12525,.T.);
#16231=ORIENTED_EDGE('',*,*,#12526,.F.);
#16232=ORIENTED_EDGE('',*,*,#12525,.F.);
#16233=ORIENTED_EDGE('',*,*,#12527,.T.);
#16234=ORIENTED_EDGE('',*,*,#12528,.T.);
#16235=ORIENTED_EDGE('',*,*,#12527,.F.);
#16236=ORIENTED_EDGE('',*,*,#12528,.F.);
#16237=ORIENTED_EDGE('',*,*,#12529,.T.);
#16238=ORIENTED_EDGE('',*,*,#12530,.T.);
#16239=ORIENTED_EDGE('',*,*,#12529,.F.);
#16240=ORIENTED_EDGE('',*,*,#12530,.F.);
#16241=ORIENTED_EDGE('',*,*,#12531,.T.);
#16242=ORIENTED_EDGE('',*,*,#12532,.F.);
#16243=ORIENTED_EDGE('',*,*,#12531,.F.);
#16244=ORIENTED_EDGE('',*,*,#12533,.T.);
#16245=ORIENTED_EDGE('',*,*,#12534,.T.);
#16246=ORIENTED_EDGE('',*,*,#12533,.F.);
#16247=ORIENTED_EDGE('',*,*,#12534,.F.);
#16248=ORIENTED_EDGE('',*,*,#12535,.T.);
#16249=ORIENTED_EDGE('',*,*,#12536,.T.);
#16250=ORIENTED_EDGE('',*,*,#12535,.F.);
#16251=ORIENTED_EDGE('',*,*,#12536,.F.);
#16252=ORIENTED_EDGE('',*,*,#12537,.T.);
#16253=ORIENTED_EDGE('',*,*,#12538,.F.);
#16254=ORIENTED_EDGE('',*,*,#12537,.F.);
#16255=ORIENTED_EDGE('',*,*,#12539,.T.);
#16256=ORIENTED_EDGE('',*,*,#12540,.T.);
#16257=ORIENTED_EDGE('',*,*,#12539,.F.);
#16258=ORIENTED_EDGE('',*,*,#12540,.F.);
#16259=ORIENTED_EDGE('',*,*,#12541,.T.);
#16260=ORIENTED_EDGE('',*,*,#12542,.T.);
#16261=ORIENTED_EDGE('',*,*,#12541,.F.);
#16262=ORIENTED_EDGE('',*,*,#12542,.F.);
#16263=ORIENTED_EDGE('',*,*,#12543,.T.);
#16264=ORIENTED_EDGE('',*,*,#12544,.F.);
#16265=ORIENTED_EDGE('',*,*,#12543,.F.);
#16266=ORIENTED_EDGE('',*,*,#12545,.T.);
#16267=ORIENTED_EDGE('',*,*,#12546,.T.);
#16268=ORIENTED_EDGE('',*,*,#12545,.F.);
#16269=ORIENTED_EDGE('',*,*,#12546,.F.);
#16270=ORIENTED_EDGE('',*,*,#12547,.T.);
#16271=ORIENTED_EDGE('',*,*,#12548,.T.);
#16272=ORIENTED_EDGE('',*,*,#12547,.F.);
#16273=ORIENTED_EDGE('',*,*,#12548,.F.);
#16274=ORIENTED_EDGE('',*,*,#12549,.T.);
#16275=ORIENTED_EDGE('',*,*,#12550,.F.);
#16276=ORIENTED_EDGE('',*,*,#12549,.F.);
#16277=ORIENTED_EDGE('',*,*,#12551,.T.);
#16278=ORIENTED_EDGE('',*,*,#12552,.T.);
#16279=ORIENTED_EDGE('',*,*,#12551,.F.);
#16280=ORIENTED_EDGE('',*,*,#12552,.F.);
#16281=ORIENTED_EDGE('',*,*,#12553,.T.);
#16282=ORIENTED_EDGE('',*,*,#12554,.T.);
#16283=ORIENTED_EDGE('',*,*,#12553,.F.);
#16284=ORIENTED_EDGE('',*,*,#12554,.F.);
#16285=ORIENTED_EDGE('',*,*,#12555,.T.);
#16286=ORIENTED_EDGE('',*,*,#12556,.F.);
#16287=ORIENTED_EDGE('',*,*,#12555,.F.);
#16288=ORIENTED_EDGE('',*,*,#12557,.T.);
#16289=ORIENTED_EDGE('',*,*,#12558,.T.);
#16290=ORIENTED_EDGE('',*,*,#12557,.F.);
#16291=ORIENTED_EDGE('',*,*,#12558,.F.);
#16292=ORIENTED_EDGE('',*,*,#12559,.T.);
#16293=ORIENTED_EDGE('',*,*,#12560,.T.);
#16294=ORIENTED_EDGE('',*,*,#12559,.F.);
#16295=ORIENTED_EDGE('',*,*,#12560,.F.);
#16296=ORIENTED_EDGE('',*,*,#12561,.T.);
#16297=ORIENTED_EDGE('',*,*,#12562,.F.);
#16298=ORIENTED_EDGE('',*,*,#12561,.F.);
#16299=ORIENTED_EDGE('',*,*,#12563,.T.);
#16300=ORIENTED_EDGE('',*,*,#12564,.T.);
#16301=ORIENTED_EDGE('',*,*,#12563,.F.);
#16302=ORIENTED_EDGE('',*,*,#12564,.F.);
#16303=ORIENTED_EDGE('',*,*,#12565,.T.);
#16304=ORIENTED_EDGE('',*,*,#12566,.T.);
#16305=ORIENTED_EDGE('',*,*,#12565,.F.);
#16306=ORIENTED_EDGE('',*,*,#12566,.F.);
#16307=ORIENTED_EDGE('',*,*,#12567,.T.);
#16308=ORIENTED_EDGE('',*,*,#12568,.F.);
#16309=ORIENTED_EDGE('',*,*,#12567,.F.);
#16310=ORIENTED_EDGE('',*,*,#12569,.T.);
#16311=ORIENTED_EDGE('',*,*,#12570,.T.);
#16312=ORIENTED_EDGE('',*,*,#12569,.F.);
#16313=ORIENTED_EDGE('',*,*,#12570,.F.);
#16314=ORIENTED_EDGE('',*,*,#12571,.T.);
#16315=ORIENTED_EDGE('',*,*,#12572,.T.);
#16316=ORIENTED_EDGE('',*,*,#12571,.F.);
#16317=ORIENTED_EDGE('',*,*,#12572,.F.);
#16318=ORIENTED_EDGE('',*,*,#12573,.T.);
#16319=ORIENTED_EDGE('',*,*,#12574,.F.);
#16320=ORIENTED_EDGE('',*,*,#12573,.F.);
#16321=ORIENTED_EDGE('',*,*,#12575,.T.);
#16322=ORIENTED_EDGE('',*,*,#12576,.T.);
#16323=ORIENTED_EDGE('',*,*,#12575,.F.);
#16324=ORIENTED_EDGE('',*,*,#12576,.F.);
#16325=ORIENTED_EDGE('',*,*,#12577,.T.);
#16326=ORIENTED_EDGE('',*,*,#12578,.T.);
#16327=ORIENTED_EDGE('',*,*,#12577,.F.);
#16328=ORIENTED_EDGE('',*,*,#12578,.F.);
#16329=ORIENTED_EDGE('',*,*,#12579,.T.);
#16330=ORIENTED_EDGE('',*,*,#12580,.F.);
#16331=ORIENTED_EDGE('',*,*,#12579,.F.);
#16332=ORIENTED_EDGE('',*,*,#12581,.T.);
#16333=ORIENTED_EDGE('',*,*,#12582,.T.);
#16334=ORIENTED_EDGE('',*,*,#12581,.F.);
#16335=ORIENTED_EDGE('',*,*,#12582,.F.);
#16336=ORIENTED_EDGE('',*,*,#12583,.T.);
#16337=ORIENTED_EDGE('',*,*,#12584,.T.);
#16338=ORIENTED_EDGE('',*,*,#12583,.F.);
#16339=ORIENTED_EDGE('',*,*,#12584,.F.);
#16340=ORIENTED_EDGE('',*,*,#12585,.T.);
#16341=ORIENTED_EDGE('',*,*,#12586,.F.);
#16342=ORIENTED_EDGE('',*,*,#12585,.F.);
#16343=ORIENTED_EDGE('',*,*,#12587,.T.);
#16344=ORIENTED_EDGE('',*,*,#12588,.T.);
#16345=ORIENTED_EDGE('',*,*,#12587,.F.);
#16346=ORIENTED_EDGE('',*,*,#12588,.F.);
#16347=ORIENTED_EDGE('',*,*,#12589,.T.);
#16348=ORIENTED_EDGE('',*,*,#12590,.T.);
#16349=ORIENTED_EDGE('',*,*,#12589,.F.);
#16350=ORIENTED_EDGE('',*,*,#12590,.F.);
#16351=ORIENTED_EDGE('',*,*,#12591,.T.);
#16352=ORIENTED_EDGE('',*,*,#12592,.F.);
#16353=ORIENTED_EDGE('',*,*,#12591,.F.);
#16354=ORIENTED_EDGE('',*,*,#12593,.T.);
#16355=ORIENTED_EDGE('',*,*,#12594,.T.);
#16356=ORIENTED_EDGE('',*,*,#12593,.F.);
#16357=ORIENTED_EDGE('',*,*,#12594,.F.);
#16358=ORIENTED_EDGE('',*,*,#12595,.T.);
#16359=ORIENTED_EDGE('',*,*,#12596,.T.);
#16360=ORIENTED_EDGE('',*,*,#12595,.F.);
#16361=ORIENTED_EDGE('',*,*,#12596,.F.);
#16362=ORIENTED_EDGE('',*,*,#12597,.T.);
#16363=ORIENTED_EDGE('',*,*,#12598,.F.);
#16364=ORIENTED_EDGE('',*,*,#12597,.F.);
#16365=ORIENTED_EDGE('',*,*,#12599,.T.);
#16366=ORIENTED_EDGE('',*,*,#12600,.T.);
#16367=ORIENTED_EDGE('',*,*,#12599,.F.);
#16368=ORIENTED_EDGE('',*,*,#12600,.F.);
#16369=ORIENTED_EDGE('',*,*,#12601,.T.);
#16370=ORIENTED_EDGE('',*,*,#12602,.T.);
#16371=ORIENTED_EDGE('',*,*,#12601,.F.);
#16372=ORIENTED_EDGE('',*,*,#12602,.F.);
#16373=ORIENTED_EDGE('',*,*,#12603,.T.);
#16374=ORIENTED_EDGE('',*,*,#12604,.F.);
#16375=ORIENTED_EDGE('',*,*,#12603,.F.);
#16376=ORIENTED_EDGE('',*,*,#12605,.T.);
#16377=ORIENTED_EDGE('',*,*,#12606,.T.);
#16378=ORIENTED_EDGE('',*,*,#12607,.T.);
#16379=ORIENTED_EDGE('',*,*,#12608,.T.);
#16380=ORIENTED_EDGE('',*,*,#12606,.F.);
#16381=ORIENTED_EDGE('',*,*,#12609,.F.);
#16382=ORIENTED_EDGE('',*,*,#12610,.F.);
#16383=ORIENTED_EDGE('',*,*,#12611,.T.);
#16384=ORIENTED_EDGE('',*,*,#12607,.F.);
#16385=ORIENTED_EDGE('',*,*,#12608,.F.);
#16386=ORIENTED_EDGE('',*,*,#12611,.F.);
#16387=ORIENTED_EDGE('',*,*,#12612,.F.);
#16388=ORIENTED_EDGE('',*,*,#12502,.T.);
#16389=ORIENTED_EDGE('',*,*,#12508,.T.);
#16390=ORIENTED_EDGE('',*,*,#12514,.T.);
#16391=ORIENTED_EDGE('',*,*,#12520,.T.);
#16392=ORIENTED_EDGE('',*,*,#12526,.T.);
#16393=ORIENTED_EDGE('',*,*,#12532,.T.);
#16394=ORIENTED_EDGE('',*,*,#12605,.F.);
#16395=ORIENTED_EDGE('',*,*,#12609,.T.);
#16396=ORIENTED_EDGE('',*,*,#12610,.T.);
#16397=ORIENTED_EDGE('',*,*,#12613,.T.);
#16398=ORIENTED_EDGE('',*,*,#12614,.T.);
#16399=ORIENTED_EDGE('',*,*,#12613,.F.);
#16400=ORIENTED_EDGE('',*,*,#12615,.F.);
#16401=ORIENTED_EDGE('',*,*,#12544,.T.);
#16402=ORIENTED_EDGE('',*,*,#12556,.T.);
#16403=ORIENTED_EDGE('',*,*,#12568,.T.);
#16404=ORIENTED_EDGE('',*,*,#12574,.T.);
#16405=ORIENTED_EDGE('',*,*,#12580,.T.);
#16406=ORIENTED_EDGE('',*,*,#12586,.T.);
#16407=ORIENTED_EDGE('',*,*,#12592,.T.);
#16408=ORIENTED_EDGE('',*,*,#12598,.T.);
#16409=ORIENTED_EDGE('',*,*,#12604,.T.);
#16410=ORIENTED_EDGE('',*,*,#12614,.F.);
#16411=ORIENTED_EDGE('',*,*,#12562,.T.);
#16412=ORIENTED_EDGE('',*,*,#12550,.T.);
#16413=ORIENTED_EDGE('',*,*,#12538,.T.);
#16414=ORIENTED_EDGE('',*,*,#12615,.T.);
#16415=ORIENTED_EDGE('',*,*,#12616,.T.);
#16416=ORIENTED_EDGE('',*,*,#12617,.T.);
#16417=ORIENTED_EDGE('',*,*,#12618,.T.);
#16418=ORIENTED_EDGE('',*,*,#12616,.F.);
#16419=ORIENTED_EDGE('',*,*,#12617,.F.);
#16420=ORIENTED_EDGE('',*,*,#12618,.F.);
#16421=ORIENTED_EDGE('',*,*,#12619,.T.);
#16422=ORIENTED_EDGE('',*,*,#12620,.F.);
#16423=ORIENTED_EDGE('',*,*,#12621,.F.);
#16424=ORIENTED_EDGE('',*,*,#12619,.F.);
#16425=ORIENTED_EDGE('',*,*,#12620,.T.);
#16426=ORIENTED_EDGE('',*,*,#12621,.T.);
#16427=ORIENTED_EDGE('',*,*,#12622,.T.);
#16428=ORIENTED_EDGE('',*,*,#12612,.T.);
#16429=ORIENTED_EDGE('',*,*,#12622,.F.);
#22995=CONICAL_SURFACE('',#24930,0.0524999999999998,1.02974425867665);
#22996=CONICAL_SURFACE('',#24934,0.155,0.78539816339745);
#22997=CONICAL_SURFACE('',#24936,0.0525000000000002,1.02974425867665);
#22998=CONICAL_SURFACE('',#24940,0.155,0.78539816339745);
#22999=CONICAL_SURFACE('',#24942,0.0525000000000002,1.02974425867665);
#23000=CONICAL_SURFACE('',#24946,0.154999999999999,0.785398163397452);
#23001=CONICAL_SURFACE('',#24948,0.0525000000000002,1.02974425867665);
#23002=CONICAL_SURFACE('',#24952,0.155,0.78539816339745);
#23003=CONICAL_SURFACE('',#24954,0.0524999999999998,1.02974425867665);
#23004=CONICAL_SURFACE('',#24958,0.155,0.78539816339745);
#23005=CONICAL_SURFACE('',#24960,0.0525000000000002,1.02974425867665);
#23006=CONICAL_SURFACE('',#24964,0.154999999999999,0.785398163397452);
#23007=CONICAL_SURFACE('',#24966,0.0525000000000002,1.02974425867665);
#23008=CONICAL_SURFACE('',#24970,0.154999999999999,0.785398163397448);
#23009=CONICAL_SURFACE('',#24972,0.0524999999999998,1.02974425867665);
#23010=CONICAL_SURFACE('',#24976,0.155,0.785398163397451);
#23011=CONICAL_SURFACE('',#24978,0.0525,1.02974425867665);
#23012=CONICAL_SURFACE('',#24982,0.155,0.785398163397451);
#23013=CONICAL_SURFACE('',#24984,0.0525,1.02974425867665);
#23014=CONICAL_SURFACE('',#24988,0.155,0.78539816339745);
#23015=CONICAL_SURFACE('',#24990,0.0525000000000002,1.02974425867665);
#23016=CONICAL_SURFACE('',#24994,0.155,0.785398163397451);
#23017=CONICAL_SURFACE('',#24996,0.0525000000000002,1.02974425867666);
#23018=CONICAL_SURFACE('',#25000,0.155,0.785398163397448);
#23019=CONICAL_SURFACE('',#25002,0.0524999999999993,1.02974425867665);
#23020=CONICAL_SURFACE('',#25006,0.155,0.785398163397453);
#23021=CONICAL_SURFACE('',#25008,0.0525000000000002,1.02974425867665);
#23022=CONICAL_SURFACE('',#25012,0.155,0.785398163397451);
#23023=CONICAL_SURFACE('',#25014,0.0525,1.02974425867665);
#23024=CONICAL_SURFACE('',#25018,0.155,0.78539816339745);
#23025=CONICAL_SURFACE('',#25020,0.0525,1.02974425867665);
#23026=CONICAL_SURFACE('',#25024,0.155,0.785398163397451);
#23027=CONICAL_SURFACE('',#25026,0.0524999999999998,1.02974425867665);
#23028=CONICAL_SURFACE('',#25030,0.155,0.785398163397448);
#23029=CONICAL_SURFACE('',#25032,0.0525000000000002,1.02974425867665);
#23030=CONICAL_SURFACE('',#25036,0.154999999999999,0.785398163397448);
#23031=CONICAL_SURFACE('',#25038,4.115,0.785398163397441);
#23032=CONICAL_SURFACE('',#25047,4.115,0.785398163397463);
#23033=CONICAL_SURFACE('',#25051,4.58,0.785398163397459);
#23034=CONICAL_SURFACE('',#25057,4.58,0.785398163397443);
#23235=ADVANCED_FACE('',(#2482),#22995,.F.);
#23236=ADVANCED_FACE('',(#2483),#1972,.F.);
#23237=ADVANCED_FACE('',(#2484),#22996,.F.);
#23238=ADVANCED_FACE('',(#2485),#22997,.F.);
#23239=ADVANCED_FACE('',(#2486),#1973,.F.);
#23240=ADVANCED_FACE('',(#2487),#22998,.F.);
#23241=ADVANCED_FACE('',(#2488),#22999,.F.);
#23242=ADVANCED_FACE('',(#2489),#1974,.F.);
#23243=ADVANCED_FACE('',(#2490),#23000,.F.);
#23244=ADVANCED_FACE('',(#2491),#23001,.F.);
#23245=ADVANCED_FACE('',(#2492),#1975,.F.);
#23246=ADVANCED_FACE('',(#2493),#23002,.F.);
#23247=ADVANCED_FACE('',(#2494),#23003,.F.);
#23248=ADVANCED_FACE('',(#2495),#1976,.F.);
#23249=ADVANCED_FACE('',(#2496),#23004,.F.);
#23250=ADVANCED_FACE('',(#2497),#23005,.F.);
#23251=ADVANCED_FACE('',(#2498),#1977,.F.);
#23252=ADVANCED_FACE('',(#2499),#23006,.F.);
#23253=ADVANCED_FACE('',(#2500),#23007,.F.);
#23254=ADVANCED_FACE('',(#2501),#1978,.F.);
#23255=ADVANCED_FACE('',(#2502),#23008,.F.);
#23256=ADVANCED_FACE('',(#2503),#23009,.F.);
#23257=ADVANCED_FACE('',(#2504),#1979,.F.);
#23258=ADVANCED_FACE('',(#2505),#23010,.F.);
#23259=ADVANCED_FACE('',(#2506),#23011,.F.);
#23260=ADVANCED_FACE('',(#2507),#1980,.F.);
#23261=ADVANCED_FACE('',(#2508),#23012,.F.);
#23262=ADVANCED_FACE('',(#2509),#23013,.F.);
#23263=ADVANCED_FACE('',(#2510),#1981,.F.);
#23264=ADVANCED_FACE('',(#2511),#23014,.F.);
#23265=ADVANCED_FACE('',(#2512),#23015,.F.);
#23266=ADVANCED_FACE('',(#2513),#1982,.F.);
#23267=ADVANCED_FACE('',(#2514),#23016,.F.);
#23268=ADVANCED_FACE('',(#2515),#23017,.F.);
#23269=ADVANCED_FACE('',(#2516),#1983,.F.);
#23270=ADVANCED_FACE('',(#2517),#23018,.F.);
#23271=ADVANCED_FACE('',(#2518),#23019,.F.);
#23272=ADVANCED_FACE('',(#2519),#1984,.F.);
#23273=ADVANCED_FACE('',(#2520),#23020,.F.);
#23274=ADVANCED_FACE('',(#2521),#23021,.F.);
#23275=ADVANCED_FACE('',(#2522),#1985,.F.);
#23276=ADVANCED_FACE('',(#2523),#23022,.F.);
#23277=ADVANCED_FACE('',(#2524),#23023,.F.);
#23278=ADVANCED_FACE('',(#2525),#1986,.F.);
#23279=ADVANCED_FACE('',(#2526),#23024,.F.);
#23280=ADVANCED_FACE('',(#2527),#23025,.F.);
#23281=ADVANCED_FACE('',(#2528),#1987,.F.);
#23282=ADVANCED_FACE('',(#2529),#23026,.F.);
#23283=ADVANCED_FACE('',(#2530),#23027,.F.);
#23284=ADVANCED_FACE('',(#2531),#1988,.F.);
#23285=ADVANCED_FACE('',(#2532),#23028,.F.);
#23286=ADVANCED_FACE('',(#2533),#23029,.F.);
#23287=ADVANCED_FACE('',(#2534),#1989,.F.);
#23288=ADVANCED_FACE('',(#2535),#23030,.F.);
#23289=ADVANCED_FACE('',(#2536),#23031,.F.);
#23290=ADVANCED_FACE('',(#2537),#1990,.F.);
#23291=ADVANCED_FACE('',(#2538,#1062,#1063,#1064,#1065,#1066,#1067,#1068),
#1287,.T.);
#23292=ADVANCED_FACE('',(#2539),#23032,.F.);
#23293=ADVANCED_FACE('',(#2540,#1069,#1070,#1071,#1072,#1073,#1074,#1075,
#1076,#1077,#1078,#1079,#1080,#1081),#1288,.T.);
#23294=ADVANCED_FACE('',(#2541),#23033,.T.);
#23295=ADVANCED_FACE('',(#2542),#1991,.T.);
#23296=ADVANCED_FACE('',(#2543),#23034,.T.);
#24530=CLOSED_SHELL('',(#23235,#23236,#23237,#23238,#23239,#23240,#23241,
#23242,#23243,#23244,#23245,#23246,#23247,#23248,#23249,#23250,#23251,#23252,
#23253,#23254,#23255,#23256,#23257,#23258,#23259,#23260,#23261,#23262,#23263,
#23264,#23265,#23266,#23267,#23268,#23269,#23270,#23271,#23272,#23273,#23274,
#23275,#23276,#23277,#23278,#23279,#23280,#23281,#23282,#23283,#23284,#23285,
#23286,#23287,#23288,#23289,#23290,#23291,#23292,#23293,#23294,#23295,#23296));
#24929=AXIS2_PLACEMENT_3D('',#34177,#27573,#27574);
#24930=AXIS2_PLACEMENT_3D('',#34178,#27575,#27576);
#24931=AXIS2_PLACEMENT_3D('',#34182,#27578,#27579);
#24932=AXIS2_PLACEMENT_3D('',#34183,#27580,#27581);
#24933=AXIS2_PLACEMENT_3D('',#34186,#27583,#27584);
#24934=AXIS2_PLACEMENT_3D('',#34187,#27585,#27586);
#24935=AXIS2_PLACEMENT_3D('',#34190,#27588,#27589);
#24936=AXIS2_PLACEMENT_3D('',#34191,#27590,#27591);
#24937=AXIS2_PLACEMENT_3D('',#34195,#27593,#27594);
#24938=AXIS2_PLACEMENT_3D('',#34196,#27595,#27596);
#24939=AXIS2_PLACEMENT_3D('',#34199,#27598,#27599);
#24940=AXIS2_PLACEMENT_3D('',#34200,#27600,#27601);
#24941=AXIS2_PLACEMENT_3D('',#34203,#27603,#27604);
#24942=AXIS2_PLACEMENT_3D('',#34204,#27605,#27606);
#24943=AXIS2_PLACEMENT_3D('',#34208,#27608,#27609);
#24944=AXIS2_PLACEMENT_3D('',#34209,#27610,#27611);
#24945=AXIS2_PLACEMENT_3D('',#34212,#27613,#27614);
#24946=AXIS2_PLACEMENT_3D('',#34213,#27615,#27616);
#24947=AXIS2_PLACEMENT_3D('',#34216,#27618,#27619);
#24948=AXIS2_PLACEMENT_3D('',#34217,#27620,#27621);
#24949=AXIS2_PLACEMENT_3D('',#34221,#27623,#27624);
#24950=AXIS2_PLACEMENT_3D('',#34222,#27625,#27626);
#24951=AXIS2_PLACEMENT_3D('',#34225,#27628,#27629);
#24952=AXIS2_PLACEMENT_3D('',#34226,#27630,#27631);
#24953=AXIS2_PLACEMENT_3D('',#34229,#27633,#27634);
#24954=AXIS2_PLACEMENT_3D('',#34230,#27635,#27636);
#24955=AXIS2_PLACEMENT_3D('',#34234,#27638,#27639);
#24956=AXIS2_PLACEMENT_3D('',#34235,#27640,#27641);
#24957=AXIS2_PLACEMENT_3D('',#34238,#27643,#27644);
#24958=AXIS2_PLACEMENT_3D('',#34239,#27645,#27646);
#24959=AXIS2_PLACEMENT_3D('',#34242,#27648,#27649);
#24960=AXIS2_PLACEMENT_3D('',#34243,#27650,#27651);
#24961=AXIS2_PLACEMENT_3D('',#34247,#27653,#27654);
#24962=AXIS2_PLACEMENT_3D('',#34248,#27655,#27656);
#24963=AXIS2_PLACEMENT_3D('',#34251,#27658,#27659);
#24964=AXIS2_PLACEMENT_3D('',#34252,#27660,#27661);
#24965=AXIS2_PLACEMENT_3D('',#34255,#27663,#27664);
#24966=AXIS2_PLACEMENT_3D('',#34256,#27665,#27666);
#24967=AXIS2_PLACEMENT_3D('',#34260,#27668,#27669);
#24968=AXIS2_PLACEMENT_3D('',#34261,#27670,#27671);
#24969=AXIS2_PLACEMENT_3D('',#34264,#27673,#27674);
#24970=AXIS2_PLACEMENT_3D('',#34265,#27675,#27676);
#24971=AXIS2_PLACEMENT_3D('',#34268,#27678,#27679);
#24972=AXIS2_PLACEMENT_3D('',#34269,#27680,#27681);
#24973=AXIS2_PLACEMENT_3D('',#34273,#27683,#27684);
#24974=AXIS2_PLACEMENT_3D('',#34274,#27685,#27686);
#24975=AXIS2_PLACEMENT_3D('',#34277,#27688,#27689);
#24976=AXIS2_PLACEMENT_3D('',#34278,#27690,#27691);
#24977=AXIS2_PLACEMENT_3D('',#34281,#27693,#27694);
#24978=AXIS2_PLACEMENT_3D('',#34282,#27695,#27696);
#24979=AXIS2_PLACEMENT_3D('',#34286,#27698,#27699);
#24980=AXIS2_PLACEMENT_3D('',#34287,#27700,#27701);
#24981=AXIS2_PLACEMENT_3D('',#34290,#27703,#27704);
#24982=AXIS2_PLACEMENT_3D('',#34291,#27705,#27706);
#24983=AXIS2_PLACEMENT_3D('',#34294,#27708,#27709);
#24984=AXIS2_PLACEMENT_3D('',#34295,#27710,#27711);
#24985=AXIS2_PLACEMENT_3D('',#34299,#27713,#27714);
#24986=AXIS2_PLACEMENT_3D('',#34300,#27715,#27716);
#24987=AXIS2_PLACEMENT_3D('',#34303,#27718,#27719);
#24988=AXIS2_PLACEMENT_3D('',#34304,#27720,#27721);
#24989=AXIS2_PLACEMENT_3D('',#34307,#27723,#27724);
#24990=AXIS2_PLACEMENT_3D('',#34308,#27725,#27726);
#24991=AXIS2_PLACEMENT_3D('',#34312,#27728,#27729);
#24992=AXIS2_PLACEMENT_3D('',#34313,#27730,#27731);
#24993=AXIS2_PLACEMENT_3D('',#34316,#27733,#27734);
#24994=AXIS2_PLACEMENT_3D('',#34317,#27735,#27736);
#24995=AXIS2_PLACEMENT_3D('',#34320,#27738,#27739);
#24996=AXIS2_PLACEMENT_3D('',#34321,#27740,#27741);
#24997=AXIS2_PLACEMENT_3D('',#34325,#27743,#27744);
#24998=AXIS2_PLACEMENT_3D('',#34326,#27745,#27746);
#24999=AXIS2_PLACEMENT_3D('',#34329,#27748,#27749);
#25000=AXIS2_PLACEMENT_3D('',#34330,#27750,#27751);
#25001=AXIS2_PLACEMENT_3D('',#34333,#27753,#27754);
#25002=AXIS2_PLACEMENT_3D('',#34334,#27755,#27756);
#25003=AXIS2_PLACEMENT_3D('',#34338,#27758,#27759);
#25004=AXIS2_PLACEMENT_3D('',#34339,#27760,#27761);
#25005=AXIS2_PLACEMENT_3D('',#34342,#27763,#27764);
#25006=AXIS2_PLACEMENT_3D('',#34343,#27765,#27766);
#25007=AXIS2_PLACEMENT_3D('',#34346,#27768,#27769);
#25008=AXIS2_PLACEMENT_3D('',#34347,#27770,#27771);
#25009=AXIS2_PLACEMENT_3D('',#34351,#27773,#27774);
#25010=AXIS2_PLACEMENT_3D('',#34352,#27775,#27776);
#25011=AXIS2_PLACEMENT_3D('',#34355,#27778,#27779);
#25012=AXIS2_PLACEMENT_3D('',#34356,#27780,#27781);
#25013=AXIS2_PLACEMENT_3D('',#34359,#27783,#27784);
#25014=AXIS2_PLACEMENT_3D('',#34360,#27785,#27786);
#25015=AXIS2_PLACEMENT_3D('',#34364,#27788,#27789);
#25016=AXIS2_PLACEMENT_3D('',#34365,#27790,#27791);
#25017=AXIS2_PLACEMENT_3D('',#34368,#27793,#27794);
#25018=AXIS2_PLACEMENT_3D('',#34369,#27795,#27796);
#25019=AXIS2_PLACEMENT_3D('',#34372,#27798,#27799);
#25020=AXIS2_PLACEMENT_3D('',#34373,#27800,#27801);
#25021=AXIS2_PLACEMENT_3D('',#34377,#27803,#27804);
#25022=AXIS2_PLACEMENT_3D('',#34378,#27805,#27806);
#25023=AXIS2_PLACEMENT_3D('',#34381,#27808,#27809);
#25024=AXIS2_PLACEMENT_3D('',#34382,#27810,#27811);
#25025=AXIS2_PLACEMENT_3D('',#34385,#27813,#27814);
#25026=AXIS2_PLACEMENT_3D('',#34386,#27815,#27816);
#25027=AXIS2_PLACEMENT_3D('',#34390,#27818,#27819);
#25028=AXIS2_PLACEMENT_3D('',#34391,#27820,#27821);
#25029=AXIS2_PLACEMENT_3D('',#34394,#27823,#27824);
#25030=AXIS2_PLACEMENT_3D('',#34395,#27825,#27826);
#25031=AXIS2_PLACEMENT_3D('',#34398,#27828,#27829);
#25032=AXIS2_PLACEMENT_3D('',#34399,#27830,#27831);
#25033=AXIS2_PLACEMENT_3D('',#34403,#27833,#27834);
#25034=AXIS2_PLACEMENT_3D('',#34404,#27835,#27836);
#25035=AXIS2_PLACEMENT_3D('',#34407,#27838,#27839);
#25036=AXIS2_PLACEMENT_3D('',#34408,#27840,#27841);
#25037=AXIS2_PLACEMENT_3D('',#34411,#27843,#27844);
#25038=AXIS2_PLACEMENT_3D('',#34412,#27845,#27846);
#25039=AXIS2_PLACEMENT_3D('',#34414,#27847,#27848);
#25040=AXIS2_PLACEMENT_3D('',#34418,#27850,#27851);
#25041=AXIS2_PLACEMENT_3D('',#34419,#27852,#27853);
#25042=AXIS2_PLACEMENT_3D('',#34420,#27854,#27855);
#25043=AXIS2_PLACEMENT_3D('',#34423,#27856,#27857);
#25044=AXIS2_PLACEMENT_3D('',#34424,#27858,#27859);
#25045=AXIS2_PLACEMENT_3D('',#34426,#27861,#27862);
#25046=AXIS2_PLACEMENT_3D('',#34428,#27863,#27864);
#25047=AXIS2_PLACEMENT_3D('',#34429,#27865,#27866);
#25048=AXIS2_PLACEMENT_3D('',#34432,#27868,#27869);
#25049=AXIS2_PLACEMENT_3D('',#34433,#27870,#27871);
#25050=AXIS2_PLACEMENT_3D('',#34435,#27872,#27873);
#25051=AXIS2_PLACEMENT_3D('',#34436,#27874,#27875);
#25052=AXIS2_PLACEMENT_3D('',#34440,#27877,#27878);
#25053=AXIS2_PLACEMENT_3D('',#34441,#27879,#27880);
#25054=AXIS2_PLACEMENT_3D('',#34442,#27881,#27882);
#25055=AXIS2_PLACEMENT_3D('',#34446,#27884,#27885);
#25056=AXIS2_PLACEMENT_3D('',#34447,#27886,#27887);
#25057=AXIS2_PLACEMENT_3D('',#34448,#27888,#27889);
#27573=DIRECTION('axis',(0.,0.,1.));
#27574=DIRECTION('refdir',(1.,0.,0.));
#27575=DIRECTION('center_axis',(0.,0.,-1.));
#27576=DIRECTION('ref_axis',(-1.,0.,0.));
#27577=DIRECTION('',(0.857167300702112,-1.04972719113862E-16,-0.515038074910055));
#27578=DIRECTION('center_axis',(0.,0.,-1.));
#27579=DIRECTION('ref_axis',(1.,0.,0.));
#27580=DIRECTION('center_axis',(0.,0.,-1.));
#27581=DIRECTION('ref_axis',(-1.,0.,0.));
#27582=DIRECTION('',(0.,0.,-1.));
#27583=DIRECTION('center_axis',(0.,0.,-1.));
#27584=DIRECTION('ref_axis',(1.,0.,0.));
#27585=DIRECTION('center_axis',(0.,0.,-1.));
#27586=DIRECTION('ref_axis',(-1.,0.,0.));
#27587=DIRECTION('',(0.707106781186548,-8.65956056235494E-17,-0.707106781186547));
#27588=DIRECTION('center_axis',(0.,0.,1.));
#27589=DIRECTION('ref_axis',(-1.,0.,0.));
#27590=DIRECTION('center_axis',(0.,0.,-1.));
#27591=DIRECTION('ref_axis',(-1.,0.,0.));
#27592=DIRECTION('',(0.857167300702112,-1.04972719113862E-16,-0.515038074910055));
#27593=DIRECTION('center_axis',(0.,0.,-1.));
#27594=DIRECTION('ref_axis',(1.,0.,0.));
#27595=DIRECTION('center_axis',(0.,0.,-1.));
#27596=DIRECTION('ref_axis',(-1.,0.,0.));
#27597=DIRECTION('',(0.,0.,-1.));
#27598=DIRECTION('center_axis',(0.,0.,-1.));
#27599=DIRECTION('ref_axis',(1.,0.,0.));
#27600=DIRECTION('center_axis',(0.,0.,-1.));
#27601=DIRECTION('ref_axis',(-1.,0.,0.));
#27602=DIRECTION('',(0.707106781186548,-8.65956056235494E-17,-0.707106781186547));
#27603=DIRECTION('center_axis',(0.,0.,1.));
#27604=DIRECTION('ref_axis',(-1.,0.,0.));
#27605=DIRECTION('center_axis',(0.,0.,-1.));
#27606=DIRECTION('ref_axis',(-1.,0.,0.));
#27607=DIRECTION('',(0.857167300702111,-1.04972719113862E-16,-0.515038074910057));
#27608=DIRECTION('center_axis',(0.,0.,-1.));
#27609=DIRECTION('ref_axis',(1.,0.,0.));
#27610=DIRECTION('center_axis',(0.,0.,-1.));
#27611=DIRECTION('ref_axis',(-1.,0.,0.));
#27612=DIRECTION('',(0.,0.,-1.));
#27613=DIRECTION('center_axis',(0.,0.,-1.));
#27614=DIRECTION('ref_axis',(1.,0.,0.));
#27615=DIRECTION('center_axis',(0.,0.,-1.));
#27616=DIRECTION('ref_axis',(-1.,0.,0.));
#27617=DIRECTION('',(0.70710678118655,-8.65956056235496E-17,-0.707106781186545));
#27618=DIRECTION('center_axis',(0.,0.,1.));
#27619=DIRECTION('ref_axis',(-1.,0.,0.));
#27620=DIRECTION('center_axis',(0.,0.,-1.));
#27621=DIRECTION('ref_axis',(-1.,0.,0.));
#27622=DIRECTION('',(0.857167300702112,-1.04972719113862E-16,-0.515038074910055));
#27623=DIRECTION('center_axis',(0.,0.,-1.));
#27624=DIRECTION('ref_axis',(1.,0.,0.));
#27625=DIRECTION('center_axis',(0.,0.,-1.));
#27626=DIRECTION('ref_axis',(-1.,0.,0.));
#27627=DIRECTION('',(0.,0.,-1.));
#27628=DIRECTION('center_axis',(0.,0.,-1.));
#27629=DIRECTION('ref_axis',(1.,0.,0.));
#27630=DIRECTION('center_axis',(0.,0.,-1.));
#27631=DIRECTION('ref_axis',(-1.,0.,0.));
#27632=DIRECTION('',(0.707106781186548,-8.65956056235494E-17,-0.707106781186547));
#27633=DIRECTION('center_axis',(0.,0.,1.));
#27634=DIRECTION('ref_axis',(-1.,0.,0.));
#27635=DIRECTION('center_axis',(0.,0.,-1.));
#27636=DIRECTION('ref_axis',(-1.,0.,0.));
#27637=DIRECTION('',(0.857167300702112,-1.04972719113862E-16,-0.515038074910055));
#27638=DIRECTION('center_axis',(0.,0.,-1.));
#27639=DIRECTION('ref_axis',(1.,0.,0.));
#27640=DIRECTION('center_axis',(0.,0.,-1.));
#27641=DIRECTION('ref_axis',(-1.,0.,0.));
#27642=DIRECTION('',(0.,0.,-1.));
#27643=DIRECTION('center_axis',(0.,0.,-1.));
#27644=DIRECTION('ref_axis',(1.,0.,0.));
#27645=DIRECTION('center_axis',(0.,0.,-1.));
#27646=DIRECTION('ref_axis',(-1.,0.,0.));
#27647=DIRECTION('',(0.707106781186548,-8.65956056235494E-17,-0.707106781186547));
#27648=DIRECTION('center_axis',(0.,0.,1.));
#27649=DIRECTION('ref_axis',(-1.,0.,0.));
#27650=DIRECTION('center_axis',(0.,0.,-1.));
#27651=DIRECTION('ref_axis',(-1.,0.,0.));
#27652=DIRECTION('',(0.857167300702111,-1.04972719113862E-16,-0.515038074910057));
#27653=DIRECTION('center_axis',(0.,0.,-1.));
#27654=DIRECTION('ref_axis',(1.,0.,0.));
#27655=DIRECTION('center_axis',(0.,0.,-1.));
#27656=DIRECTION('ref_axis',(-1.,0.,0.));
#27657=DIRECTION('',(0.,0.,-1.));
#27658=DIRECTION('center_axis',(0.,0.,-1.));
#27659=DIRECTION('ref_axis',(1.,0.,0.));
#27660=DIRECTION('center_axis',(0.,0.,-1.));
#27661=DIRECTION('ref_axis',(-1.,0.,0.));
#27662=DIRECTION('',(0.70710678118655,-8.65956056235496E-17,-0.707106781186545));
#27663=DIRECTION('center_axis',(0.,0.,1.));
#27664=DIRECTION('ref_axis',(-1.,0.,0.));
#27665=DIRECTION('center_axis',(0.,0.,1.));
#27666=DIRECTION('ref_axis',(1.,0.,0.));
#27667=DIRECTION('',(-0.857167300702111,-1.04972719113862E-16,0.515038074910057));
#27668=DIRECTION('center_axis',(0.,0.,1.));
#27669=DIRECTION('ref_axis',(1.,0.,0.));
#27670=DIRECTION('center_axis',(0.,0.,1.));
#27671=DIRECTION('ref_axis',(1.,0.,0.));
#27672=DIRECTION('',(0.,0.,1.));
#27673=DIRECTION('center_axis',(0.,0.,1.));
#27674=DIRECTION('ref_axis',(1.,0.,0.));
#27675=DIRECTION('center_axis',(0.,0.,1.));
#27676=DIRECTION('ref_axis',(1.,0.,0.));
#27677=DIRECTION('',(-0.707106781186547,-8.65956056235493E-17,0.707106781186547));
#27678=DIRECTION('center_axis',(0.,0.,-1.));
#27679=DIRECTION('ref_axis',(1.,0.,0.));
#27680=DIRECTION('center_axis',(0.,0.,1.));
#27681=DIRECTION('ref_axis',(1.,0.,0.));
#27682=DIRECTION('',(-0.857167300702112,-1.04972719113862E-16,0.515038074910055));
#27683=DIRECTION('center_axis',(0.,0.,1.));
#27684=DIRECTION('ref_axis',(1.,0.,0.));
#27685=DIRECTION('center_axis',(0.,0.,1.));
#27686=DIRECTION('ref_axis',(1.,0.,0.));
#27687=DIRECTION('',(0.,0.,1.));
#27688=DIRECTION('center_axis',(0.,0.,1.));
#27689=DIRECTION('ref_axis',(1.,0.,0.));
#27690=DIRECTION('center_axis',(0.,0.,1.));
#27691=DIRECTION('ref_axis',(1.,0.,0.));
#27692=DIRECTION('',(-0.707106781186549,-8.65956056235495E-17,0.707106781186546));
#27693=DIRECTION('center_axis',(0.,0.,-1.));
#27694=DIRECTION('ref_axis',(1.,0.,0.));
#27695=DIRECTION('center_axis',(0.,0.,1.));
#27696=DIRECTION('ref_axis',(1.,0.,0.));
#27697=DIRECTION('',(-0.857167300702112,-1.04972719113862E-16,0.515038074910055));
#27698=DIRECTION('center_axis',(0.,0.,1.));
#27699=DIRECTION('ref_axis',(1.,0.,0.));
#27700=DIRECTION('center_axis',(0.,0.,1.));
#27701=DIRECTION('ref_axis',(1.,0.,0.));
#27702=DIRECTION('',(0.,0.,1.));
#27703=DIRECTION('center_axis',(0.,0.,1.));
#27704=DIRECTION('ref_axis',(1.,0.,0.));
#27705=DIRECTION('center_axis',(0.,0.,1.));
#27706=DIRECTION('ref_axis',(1.,0.,0.));
#27707=DIRECTION('',(-0.707106781186549,-8.65956056235495E-17,0.707106781186546));
#27708=DIRECTION('center_axis',(0.,0.,-1.));
#27709=DIRECTION('ref_axis',(1.,0.,0.));
#27710=DIRECTION('center_axis',(0.,0.,1.));
#27711=DIRECTION('ref_axis',(1.,0.,0.));
#27712=DIRECTION('',(-0.857167300702112,-1.04972719113862E-16,0.515038074910055));
#27713=DIRECTION('center_axis',(0.,0.,1.));
#27714=DIRECTION('ref_axis',(1.,0.,0.));
#27715=DIRECTION('center_axis',(0.,0.,1.));
#27716=DIRECTION('ref_axis',(1.,0.,0.));
#27717=DIRECTION('',(0.,0.,1.));
#27718=DIRECTION('center_axis',(0.,0.,1.));
#27719=DIRECTION('ref_axis',(1.,0.,0.));
#27720=DIRECTION('center_axis',(0.,0.,1.));
#27721=DIRECTION('ref_axis',(1.,0.,0.));
#27722=DIRECTION('',(-0.707106781186549,-8.65956056235495E-17,0.707106781186546));
#27723=DIRECTION('center_axis',(0.,0.,-1.));
#27724=DIRECTION('ref_axis',(1.,0.,0.));
#27725=DIRECTION('center_axis',(0.,0.,1.));
#27726=DIRECTION('ref_axis',(1.,0.,0.));
#27727=DIRECTION('',(-0.857167300702112,-1.04972719113862E-16,0.515038074910055));
#27728=DIRECTION('center_axis',(0.,0.,1.));
#27729=DIRECTION('ref_axis',(1.,0.,0.));
#27730=DIRECTION('center_axis',(0.,0.,1.));
#27731=DIRECTION('ref_axis',(1.,0.,0.));
#27732=DIRECTION('',(0.,0.,1.));
#27733=DIRECTION('center_axis',(0.,0.,1.));
#27734=DIRECTION('ref_axis',(1.,0.,0.));
#27735=DIRECTION('center_axis',(0.,0.,1.));
#27736=DIRECTION('ref_axis',(1.,0.,0.));
#27737=DIRECTION('',(-0.707106781186549,-8.65956056235495E-17,0.707106781186546));
#27738=DIRECTION('center_axis',(0.,0.,-1.));
#27739=DIRECTION('ref_axis',(1.,0.,0.));
#27740=DIRECTION('center_axis',(0.,0.,1.));
#27741=DIRECTION('ref_axis',(1.,0.,0.));
#27742=DIRECTION('',(-0.857167300702113,-1.04972719113862E-16,0.515038074910054));
#27743=DIRECTION('center_axis',(0.,0.,1.));
#27744=DIRECTION('ref_axis',(1.,0.,0.));
#27745=DIRECTION('center_axis',(0.,0.,1.));
#27746=DIRECTION('ref_axis',(1.,0.,0.));
#27747=DIRECTION('',(0.,0.,1.));
#27748=DIRECTION('center_axis',(0.,0.,1.));
#27749=DIRECTION('ref_axis',(1.,0.,0.));
#27750=DIRECTION('center_axis',(0.,0.,1.));
#27751=DIRECTION('ref_axis',(1.,0.,0.));
#27752=DIRECTION('',(-0.707106781186548,-8.65956056235494E-17,0.707106781186548));
#27753=DIRECTION('center_axis',(0.,0.,-1.));
#27754=DIRECTION('ref_axis',(1.,0.,0.));
#27755=DIRECTION('center_axis',(0.,0.,1.));
#27756=DIRECTION('ref_axis',(1.,0.,0.));
#27757=DIRECTION('',(-0.857167300702111,-1.04972719113862E-16,0.515038074910057));
#27758=DIRECTION('center_axis',(0.,0.,1.));
#27759=DIRECTION('ref_axis',(1.,0.,0.));
#27760=DIRECTION('center_axis',(0.,0.,1.));
#27761=DIRECTION('ref_axis',(1.,0.,0.));
#27762=DIRECTION('',(0.,0.,1.));
#27763=DIRECTION('center_axis',(0.,0.,1.));
#27764=DIRECTION('ref_axis',(1.,0.,0.));
#27765=DIRECTION('center_axis',(0.,0.,1.));
#27766=DIRECTION('ref_axis',(1.,0.,0.));
#27767=DIRECTION('',(-0.707106781186551,-8.65956056235497E-17,0.707106781186544));
#27768=DIRECTION('center_axis',(0.,0.,-1.));
#27769=DIRECTION('ref_axis',(1.,0.,0.));
#27770=DIRECTION('center_axis',(0.,0.,1.));
#27771=DIRECTION('ref_axis',(1.,0.,0.));
#27772=DIRECTION('',(-0.857167300702112,-1.04972719113862E-16,0.515038074910055));
#27773=DIRECTION('center_axis',(0.,0.,1.));
#27774=DIRECTION('ref_axis',(1.,0.,0.));
#27775=DIRECTION('center_axis',(0.,0.,1.));
#27776=DIRECTION('ref_axis',(1.,0.,0.));
#27777=DIRECTION('',(0.,0.,1.));
#27778=DIRECTION('center_axis',(0.,0.,1.));
#27779=DIRECTION('ref_axis',(1.,0.,0.));
#27780=DIRECTION('center_axis',(0.,0.,1.));
#27781=DIRECTION('ref_axis',(1.,0.,0.));
#27782=DIRECTION('',(-0.707106781186549,-8.65956056235495E-17,0.707106781186546));
#27783=DIRECTION('center_axis',(0.,0.,-1.));
#27784=DIRECTION('ref_axis',(1.,0.,0.));
#27785=DIRECTION('center_axis',(0.,0.,1.));
#27786=DIRECTION('ref_axis',(1.,0.,0.));
#27787=DIRECTION('',(-0.857167300702112,-1.04972719113862E-16,0.515038074910055));
#27788=DIRECTION('center_axis',(0.,0.,1.));
#27789=DIRECTION('ref_axis',(1.,0.,0.));
#27790=DIRECTION('center_axis',(0.,0.,1.));
#27791=DIRECTION('ref_axis',(1.,0.,0.));
#27792=DIRECTION('',(0.,0.,1.));
#27793=DIRECTION('center_axis',(0.,0.,1.));
#27794=DIRECTION('ref_axis',(1.,0.,0.));
#27795=DIRECTION('center_axis',(0.,0.,1.));
#27796=DIRECTION('ref_axis',(1.,0.,0.));
#27797=DIRECTION('',(-0.707106781186548,-8.65956056235494E-17,0.707106781186547));
#27798=DIRECTION('center_axis',(0.,0.,-1.));
#27799=DIRECTION('ref_axis',(1.,0.,0.));
#27800=DIRECTION('center_axis',(0.,0.,1.));
#27801=DIRECTION('ref_axis',(1.,0.,0.));
#27802=DIRECTION('',(-0.857167300702112,-1.04972719113862E-16,0.515038074910055));
#27803=DIRECTION('center_axis',(0.,0.,1.));
#27804=DIRECTION('ref_axis',(1.,0.,0.));
#27805=DIRECTION('center_axis',(0.,0.,1.));
#27806=DIRECTION('ref_axis',(1.,0.,0.));
#27807=DIRECTION('',(0.,0.,1.));
#27808=DIRECTION('center_axis',(0.,0.,1.));
#27809=DIRECTION('ref_axis',(1.,0.,0.));
#27810=DIRECTION('center_axis',(0.,0.,1.));
#27811=DIRECTION('ref_axis',(1.,0.,0.));
#27812=DIRECTION('',(-0.707106781186549,-8.65956056235495E-17,0.707106781186546));
#27813=DIRECTION('center_axis',(0.,0.,-1.));
#27814=DIRECTION('ref_axis',(1.,0.,0.));
#27815=DIRECTION('center_axis',(0.,0.,1.));
#27816=DIRECTION('ref_axis',(1.,0.,0.));
#27817=DIRECTION('',(-0.857167300702112,-1.04972719113862E-16,0.515038074910055));
#27818=DIRECTION('center_axis',(0.,0.,1.));
#27819=DIRECTION('ref_axis',(1.,0.,0.));
#27820=DIRECTION('center_axis',(0.,0.,1.));
#27821=DIRECTION('ref_axis',(1.,0.,0.));
#27822=DIRECTION('',(0.,0.,1.));
#27823=DIRECTION('center_axis',(0.,0.,1.));
#27824=DIRECTION('ref_axis',(1.,0.,0.));
#27825=DIRECTION('center_axis',(0.,0.,1.));
#27826=DIRECTION('ref_axis',(1.,0.,0.));
#27827=DIRECTION('',(-0.707106781186547,-8.65956056235493E-17,0.707106781186547));
#27828=DIRECTION('center_axis',(0.,0.,-1.));
#27829=DIRECTION('ref_axis',(1.,0.,0.));
#27830=DIRECTION('center_axis',(0.,0.,1.));
#27831=DIRECTION('ref_axis',(1.,0.,0.));
#27832=DIRECTION('',(-0.857167300702111,-1.04972719113862E-16,0.515038074910057));
#27833=DIRECTION('center_axis',(0.,0.,1.));
#27834=DIRECTION('ref_axis',(1.,0.,0.));
#27835=DIRECTION('center_axis',(0.,0.,1.));
#27836=DIRECTION('ref_axis',(1.,0.,0.));
#27837=DIRECTION('',(0.,0.,1.));
#27838=DIRECTION('center_axis',(0.,0.,1.));
#27839=DIRECTION('ref_axis',(1.,0.,0.));
#27840=DIRECTION('center_axis',(0.,0.,1.));
#27841=DIRECTION('ref_axis',(1.,0.,0.));
#27842=DIRECTION('',(-0.707106781186547,-8.65956056235493E-17,0.707106781186547));
#27843=DIRECTION('center_axis',(0.,0.,-1.));
#27844=DIRECTION('ref_axis',(1.,0.,0.));
#27845=DIRECTION('center_axis',(0.,0.,-1.));
#27846=DIRECTION('ref_axis',(-1.,0.,0.));
#27847=DIRECTION('center_axis',(0.,0.,-1.));
#27848=DIRECTION('ref_axis',(-1.,0.,0.));
#27849=DIRECTION('',(-0.707106781186542,8.65956056235487E-17,0.707106781186553));
#27850=DIRECTION('center_axis',(0.,0.,1.));
#27851=DIRECTION('ref_axis',(-1.,0.,0.));
#27852=DIRECTION('center_axis',(0.,0.,1.));
#27853=DIRECTION('ref_axis',(-1.,0.,0.));
#27854=DIRECTION('center_axis',(0.,0.,1.));
#27855=DIRECTION('ref_axis',(1.,0.,0.));
#27856=DIRECTION('center_axis',(0.,0.,-1.));
#27857=DIRECTION('ref_axis',(-1.,0.,0.));
#27858=DIRECTION('center_axis',(0.,0.,-1.));
#27859=DIRECTION('ref_axis',(-1.,0.,0.));
#27860=DIRECTION('',(0.,0.,-1.));
#27861=DIRECTION('center_axis',(0.,0.,-1.));
#27862=DIRECTION('ref_axis',(-1.,0.,0.));
#27863=DIRECTION('center_axis',(0.,0.,1.));
#27864=DIRECTION('ref_axis',(-1.,0.,0.));
#27865=DIRECTION('center_axis',(0.,0.,1.));
#27866=DIRECTION('ref_axis',(-1.,0.,0.));
#27867=DIRECTION('',(0.707106781186558,-8.65956056235506E-17,0.707106781186537));
#27868=DIRECTION('center_axis',(0.,0.,1.));
#27869=DIRECTION('ref_axis',(-1.,0.,0.));
#27870=DIRECTION('center_axis',(0.,0.,1.));
#27871=DIRECTION('ref_axis',(1.,0.,0.));
#27872=DIRECTION('center_axis',(0.,0.,-1.));
#27873=DIRECTION('ref_axis',(-1.,0.,0.));
#27874=DIRECTION('center_axis',(0.,0.,-1.));
#27875=DIRECTION('ref_axis',(-1.,0.,0.));
#27876=DIRECTION('',(0.707106781186555,8.65956056235503E-17,-0.70710678118654));
#27877=DIRECTION('center_axis',(0.,0.,1.));
#27878=DIRECTION('ref_axis',(-1.,0.,0.));
#27879=DIRECTION('center_axis',(0.,0.,1.));
#27880=DIRECTION('ref_axis',(-1.,0.,0.));
#27881=DIRECTION('center_axis',(0.,0.,1.));
#27882=DIRECTION('ref_axis',(1.,0.,0.));
#27883=DIRECTION('',(0.,0.,-1.));
#27884=DIRECTION('center_axis',(0.,0.,-1.));
#27885=DIRECTION('ref_axis',(-1.,0.,0.));
#27886=DIRECTION('center_axis',(0.,0.,-1.));
#27887=DIRECTION('ref_axis',(-1.,0.,0.));
#27888=DIRECTION('center_axis',(0.,0.,1.));
#27889=DIRECTION('ref_axis',(-1.,0.,0.));
#27890=DIRECTION('',(-0.707106781186544,-8.65956056235488E-17,-0.707106781186551));
#34177=CARTESIAN_POINT('',(0.,0.,0.));
#34178=CARTESIAN_POINT('Origin',(2.16,-3.74122974434878,2.23154518249895));
#34179=CARTESIAN_POINT('',(2.16,-3.74122974434878,2.26309036499789));
#34180=CARTESIAN_POINT('',(2.265,-3.74122974434878,2.2));
#34181=CARTESIAN_POINT('',(2.2125,-3.74122974434878,2.23154518249895));
#34182=CARTESIAN_POINT('Origin',(2.16,-3.74122974434878,2.2));
#34183=CARTESIAN_POINT('Origin',(2.16,-3.74122974434878,1.825));
#34184=CARTESIAN_POINT('',(2.265,-3.74122974434878,1.45));
#34185=CARTESIAN_POINT('',(2.265,-3.74122974434878,1.825));
#34186=CARTESIAN_POINT('Origin',(2.16,-3.74122974434878,1.45));
#34187=CARTESIAN_POINT('Origin',(2.16,-3.74122974434878,1.4));
#34188=CARTESIAN_POINT('',(2.315,-3.74122974434878,1.4));
#34189=CARTESIAN_POINT('',(2.315,-3.74122974434878,1.4));
#34190=CARTESIAN_POINT('Origin',(2.16,-3.74122974434878,1.4));
#34191=CARTESIAN_POINT('Origin',(-2.16,-3.74122974434877,2.23154518249895));
#34192=CARTESIAN_POINT('',(-2.16,-3.74122974434877,2.26309036499789));
#34193=CARTESIAN_POINT('',(-2.055,-3.74122974434877,2.2));
#34194=CARTESIAN_POINT('',(-2.1075,-3.74122974434877,2.23154518249895));
#34195=CARTESIAN_POINT('Origin',(-2.16,-3.74122974434877,2.2));
#34196=CARTESIAN_POINT('Origin',(-2.16,-3.74122974434877,1.825));
#34197=CARTESIAN_POINT('',(-2.055,-3.74122974434877,1.45));
#34198=CARTESIAN_POINT('',(-2.055,-3.74122974434877,1.825));
#34199=CARTESIAN_POINT('Origin',(-2.16,-3.74122974434877,1.45));
#34200=CARTESIAN_POINT('Origin',(-2.16,-3.74122974434877,1.4));
#34201=CARTESIAN_POINT('',(-2.005,-3.74122974434877,1.4));
#34202=CARTESIAN_POINT('',(-2.005,-3.74122974434877,1.4));
#34203=CARTESIAN_POINT('Origin',(-2.16,-3.74122974434877,1.4));
#34204=CARTESIAN_POINT('Origin',(-4.32,5.29047417231657E-16,2.23154518249895));
#34205=CARTESIAN_POINT('',(-4.32,5.29047417231657E-16,2.26309036499789));
#34206=CARTESIAN_POINT('',(-4.215,5.16188625840609E-16,2.2));
#34207=CARTESIAN_POINT('',(-4.2675,5.22618021536133E-16,2.23154518249895));
#34208=CARTESIAN_POINT('Origin',(-4.32,5.29047417231657E-16,2.2));
#34209=CARTESIAN_POINT('Origin',(-4.32,5.29047417231657E-16,1.825));
#34210=CARTESIAN_POINT('',(-4.215,5.16188625840609E-16,1.45));
#34211=CARTESIAN_POINT('',(-4.215,5.16188625840609E-16,1.825));
#34212=CARTESIAN_POINT('Origin',(-4.32,5.29047417231657E-16,1.45));
#34213=CARTESIAN_POINT('Origin',(-4.32,5.29047417231657E-16,1.4));
#34214=CARTESIAN_POINT('',(-4.165,5.48029442618441E-16,1.4));
#34215=CARTESIAN_POINT('',(-4.165,5.10065391844873E-16,1.4));
#34216=CARTESIAN_POINT('Origin',(-4.32,5.29047417231657E-16,1.4));
#34217=CARTESIAN_POINT('Origin',(-2.16,3.74122974434878,2.23154518249895));
#34218=CARTESIAN_POINT('',(-2.16,3.74122974434878,2.26309036499789));
#34219=CARTESIAN_POINT('',(-2.055,3.74122974434878,2.2));
#34220=CARTESIAN_POINT('',(-2.1075,3.74122974434878,2.23154518249895));
#34221=CARTESIAN_POINT('Origin',(-2.16,3.74122974434878,2.2));
#34222=CARTESIAN_POINT('Origin',(-2.16,3.74122974434878,1.825));
#34223=CARTESIAN_POINT('',(-2.055,3.74122974434878,1.45));
#34224=CARTESIAN_POINT('',(-2.055,3.74122974434878,1.825));
#34225=CARTESIAN_POINT('Origin',(-2.16,3.74122974434878,1.45));
#34226=CARTESIAN_POINT('Origin',(-2.16,3.74122974434878,1.4));
#34227=CARTESIAN_POINT('',(-2.005,3.74122974434878,1.4));
#34228=CARTESIAN_POINT('',(-2.005,3.74122974434878,1.4));
#34229=CARTESIAN_POINT('Origin',(-2.16,3.74122974434878,1.4));
#34230=CARTESIAN_POINT('Origin',(2.16,3.74122974434878,2.23154518249895));
#34231=CARTESIAN_POINT('',(2.16,3.74122974434878,2.26309036499789));
#34232=CARTESIAN_POINT('',(2.265,3.74122974434878,2.2));
#34233=CARTESIAN_POINT('',(2.2125,3.74122974434878,2.23154518249895));
#34234=CARTESIAN_POINT('Origin',(2.16,3.74122974434878,2.2));
#34235=CARTESIAN_POINT('Origin',(2.16,3.74122974434878,1.825));
#34236=CARTESIAN_POINT('',(2.265,3.74122974434878,1.45));
#34237=CARTESIAN_POINT('',(2.265,3.74122974434878,1.825));
#34238=CARTESIAN_POINT('Origin',(2.16,3.74122974434878,1.45));
#34239=CARTESIAN_POINT('Origin',(2.16,3.74122974434878,1.4));
#34240=CARTESIAN_POINT('',(2.315,3.74122974434878,1.4));
#34241=CARTESIAN_POINT('',(2.315,3.74122974434878,1.4));
#34242=CARTESIAN_POINT('Origin',(2.16,3.74122974434878,1.4));
#34243=CARTESIAN_POINT('Origin',(4.32,0.,2.23154518249895));
#34244=CARTESIAN_POINT('',(4.32,0.,2.26309036499789));
#34245=CARTESIAN_POINT('',(4.425,-1.28587913910472E-17,2.2));
#34246=CARTESIAN_POINT('',(4.3725,-6.42939569552363E-18,2.23154518249895));
#34247=CARTESIAN_POINT('Origin',(4.32,0.,2.2));
#34248=CARTESIAN_POINT('Origin',(4.32,0.,1.825));
#34249=CARTESIAN_POINT('',(4.425,-1.28587913910472E-17,1.45));
#34250=CARTESIAN_POINT('',(4.425,-1.28587913910472E-17,1.825));
#34251=CARTESIAN_POINT('Origin',(4.32,0.,1.45));
#34252=CARTESIAN_POINT('Origin',(4.32,0.,1.4));
#34253=CARTESIAN_POINT('',(4.475,1.89820253867839E-17,1.4));
#34254=CARTESIAN_POINT('',(4.475,-1.89820253867839E-17,1.4));
#34255=CARTESIAN_POINT('Origin',(4.32,0.,1.4));
#34256=CARTESIAN_POINT('Origin',(4.17279956956878,-1.11809827484289,10.3684548175011));
#34257=CARTESIAN_POINT('',(4.17279956956878,-1.11809827484289,10.3369096350021));
#34258=CARTESIAN_POINT('',(4.06779956956878,-1.11809827484289,10.4));
#34259=CARTESIAN_POINT('',(4.12029956956878,-1.11809827484289,10.3684548175011));
#34260=CARTESIAN_POINT('Origin',(4.17279956956878,-1.11809827484289,10.4));
#34261=CARTESIAN_POINT('Origin',(4.17279956956878,-1.11809827484289,10.875));
#34262=CARTESIAN_POINT('',(4.06779956956878,-1.11809827484289,11.35));
#34263=CARTESIAN_POINT('',(4.06779956956878,-1.11809827484289,10.875));
#34264=CARTESIAN_POINT('Origin',(4.17279956956878,-1.11809827484289,11.35));
#34265=CARTESIAN_POINT('Origin',(4.17279956956878,-1.11809827484289,11.4));
#34266=CARTESIAN_POINT('',(4.01779956956878,-1.11809827484289,11.4));
#34267=CARTESIAN_POINT('',(4.01779956956878,-1.11809827484289,11.4));
#34268=CARTESIAN_POINT('Origin',(4.17279956956878,-1.11809827484289,11.4));
#34269=CARTESIAN_POINT('Origin',(3.05470129472588,-3.05470129472589,10.3684548175011));
#34270=CARTESIAN_POINT('',(3.05470129472588,-3.05470129472589,10.3369096350021));
#34271=CARTESIAN_POINT('',(2.94970129472588,-3.05470129472589,10.4));
#34272=CARTESIAN_POINT('',(3.00220129472588,-3.05470129472589,10.3684548175011));
#34273=CARTESIAN_POINT('Origin',(3.05470129472588,-3.05470129472589,10.4));
#34274=CARTESIAN_POINT('Origin',(3.05470129472588,-3.05470129472589,10.875));
#34275=CARTESIAN_POINT('',(2.94970129472588,-3.05470129472589,11.35));
#34276=CARTESIAN_POINT('',(2.94970129472588,-3.05470129472589,10.875));
#34277=CARTESIAN_POINT('Origin',(3.05470129472588,-3.05470129472589,11.35));
#34278=CARTESIAN_POINT('Origin',(3.05470129472588,-3.05470129472589,11.4));
#34279=CARTESIAN_POINT('',(2.89970129472588,-3.05470129472589,11.4));
#34280=CARTESIAN_POINT('',(2.89970129472588,-3.05470129472589,11.4));
#34281=CARTESIAN_POINT('Origin',(3.05470129472588,-3.05470129472589,11.4));
#34282=CARTESIAN_POINT('Origin',(1.11809827484289,-4.17279956956878,10.3684548175011));
#34283=CARTESIAN_POINT('',(1.11809827484289,-4.17279956956878,10.3369096350021));
#34284=CARTESIAN_POINT('',(1.01309827484289,-4.17279956956878,10.4));
#34285=CARTESIAN_POINT('',(1.06559827484289,-4.17279956956878,10.3684548175011));
#34286=CARTESIAN_POINT('Origin',(1.11809827484289,-4.17279956956878,10.4));
#34287=CARTESIAN_POINT('Origin',(1.11809827484289,-4.17279956956878,10.875));
#34288=CARTESIAN_POINT('',(1.01309827484289,-4.17279956956878,11.35));
#34289=CARTESIAN_POINT('',(1.01309827484289,-4.17279956956878,10.875));
#34290=CARTESIAN_POINT('Origin',(1.11809827484289,-4.17279956956878,11.35));
#34291=CARTESIAN_POINT('Origin',(1.11809827484289,-4.17279956956878,11.4));
#34292=CARTESIAN_POINT('',(0.963098274842888,-4.17279956956878,11.4));
#34293=CARTESIAN_POINT('',(0.963098274842888,-4.17279956956878,11.4));
#34294=CARTESIAN_POINT('Origin',(1.11809827484289,-4.17279956956878,11.4));
#34295=CARTESIAN_POINT('Origin',(-1.11809827484289,-4.17279956956878,10.3684548175011));
#34296=CARTESIAN_POINT('',(-1.11809827484289,-4.17279956956878,10.3369096350021));
#34297=CARTESIAN_POINT('',(-1.22309827484289,-4.17279956956878,10.4));
#34298=CARTESIAN_POINT('',(-1.17059827484289,-4.17279956956878,10.3684548175011));
#34299=CARTESIAN_POINT('Origin',(-1.11809827484289,-4.17279956956878,10.4));
#34300=CARTESIAN_POINT('Origin',(-1.11809827484289,-4.17279956956878,10.875));
#34301=CARTESIAN_POINT('',(-1.22309827484289,-4.17279956956878,11.35));
#34302=CARTESIAN_POINT('',(-1.22309827484289,-4.17279956956878,10.875));
#34303=CARTESIAN_POINT('Origin',(-1.11809827484289,-4.17279956956878,11.35));
#34304=CARTESIAN_POINT('Origin',(-1.11809827484289,-4.17279956956878,11.4));
#34305=CARTESIAN_POINT('',(-1.27309827484289,-4.17279956956878,11.4));
#34306=CARTESIAN_POINT('',(-1.27309827484289,-4.17279956956878,11.4));
#34307=CARTESIAN_POINT('Origin',(-1.11809827484289,-4.17279956956878,11.4));
#34308=CARTESIAN_POINT('Origin',(-3.05470129472589,-3.05470129472589,10.3684548175011));
#34309=CARTESIAN_POINT('',(-3.05470129472589,-3.05470129472589,10.3369096350021));
#34310=CARTESIAN_POINT('',(-3.15970129472589,-3.05470129472589,10.4));
#34311=CARTESIAN_POINT('',(-3.10720129472589,-3.05470129472589,10.3684548175011));
#34312=CARTESIAN_POINT('Origin',(-3.05470129472589,-3.05470129472589,10.4));
#34313=CARTESIAN_POINT('Origin',(-3.05470129472589,-3.05470129472589,10.875));
#34314=CARTESIAN_POINT('',(-3.15970129472589,-3.05470129472589,11.35));
#34315=CARTESIAN_POINT('',(-3.15970129472589,-3.05470129472589,10.875));
#34316=CARTESIAN_POINT('Origin',(-3.05470129472589,-3.05470129472589,11.35));
#34317=CARTESIAN_POINT('Origin',(-3.05470129472589,-3.05470129472589,11.4));
#34318=CARTESIAN_POINT('',(-3.20970129472589,-3.05470129472589,11.4));
#34319=CARTESIAN_POINT('',(-3.20970129472589,-3.05470129472589,11.4));
#34320=CARTESIAN_POINT('Origin',(-3.05470129472589,-3.05470129472589,11.4));
#34321=CARTESIAN_POINT('Origin',(-4.17279956956878,-1.11809827484289,10.3684548175011));
#34322=CARTESIAN_POINT('',(-4.17279956956878,-1.11809827484289,10.3369096350021));
#34323=CARTESIAN_POINT('',(-4.27779956956878,-1.11809827484289,10.4));
#34324=CARTESIAN_POINT('',(-4.22529956956878,-1.11809827484289,10.3684548175011));
#34325=CARTESIAN_POINT('Origin',(-4.17279956956878,-1.11809827484289,10.4));
#34326=CARTESIAN_POINT('Origin',(-4.17279956956878,-1.11809827484289,10.875));
#34327=CARTESIAN_POINT('',(-4.27779956956878,-1.11809827484289,11.35));
#34328=CARTESIAN_POINT('',(-4.27779956956878,-1.11809827484289,10.875));
#34329=CARTESIAN_POINT('Origin',(-4.17279956956878,-1.11809827484289,11.35));
#34330=CARTESIAN_POINT('Origin',(-4.17279956956878,-1.11809827484289,11.4));
#34331=CARTESIAN_POINT('',(-4.32779956956878,-1.11809827484289,11.4));
#34332=CARTESIAN_POINT('',(-4.32779956956878,-1.11809827484289,11.4));
#34333=CARTESIAN_POINT('Origin',(-4.17279956956878,-1.11809827484289,11.4));
#34334=CARTESIAN_POINT('Origin',(-4.17279956956877,1.11809827484289,10.3684548175011));
#34335=CARTESIAN_POINT('',(-4.17279956956877,1.11809827484289,10.3369096350021));
#34336=CARTESIAN_POINT('',(-4.27779956956877,1.11809827484289,10.4));
#34337=CARTESIAN_POINT('',(-4.22529956956877,1.11809827484289,10.3684548175011));
#34338=CARTESIAN_POINT('Origin',(-4.17279956956877,1.11809827484289,10.4));
#34339=CARTESIAN_POINT('Origin',(-4.17279956956877,1.11809827484289,10.875));
#34340=CARTESIAN_POINT('',(-4.27779956956877,1.11809827484289,11.35));
#34341=CARTESIAN_POINT('',(-4.27779956956877,1.11809827484289,10.875));
#34342=CARTESIAN_POINT('Origin',(-4.17279956956877,1.11809827484289,11.35));
#34343=CARTESIAN_POINT('Origin',(-4.17279956956877,1.11809827484289,11.4));
#34344=CARTESIAN_POINT('',(-4.32779956956877,1.11809827484289,11.4));
#34345=CARTESIAN_POINT('',(-4.32779956956877,1.11809827484289,11.4));
#34346=CARTESIAN_POINT('Origin',(-4.17279956956877,1.11809827484289,11.4));
#34347=CARTESIAN_POINT('Origin',(-3.05470129472589,3.05470129472589,10.3684548175011));
#34348=CARTESIAN_POINT('',(-3.05470129472589,3.05470129472589,10.3369096350021));
#34349=CARTESIAN_POINT('',(-3.15970129472589,3.05470129472589,10.4));
#34350=CARTESIAN_POINT('',(-3.10720129472589,3.05470129472589,10.3684548175011));
#34351=CARTESIAN_POINT('Origin',(-3.05470129472589,3.05470129472589,10.4));
#34352=CARTESIAN_POINT('Origin',(-3.05470129472589,3.05470129472589,10.875));
#34353=CARTESIAN_POINT('',(-3.15970129472589,3.05470129472589,11.35));
#34354=CARTESIAN_POINT('',(-3.15970129472589,3.05470129472589,10.875));
#34355=CARTESIAN_POINT('Origin',(-3.05470129472589,3.05470129472589,11.35));
#34356=CARTESIAN_POINT('Origin',(-3.05470129472589,3.05470129472589,11.4));
#34357=CARTESIAN_POINT('',(-3.20970129472589,3.05470129472589,11.4));
#34358=CARTESIAN_POINT('',(-3.20970129472589,3.05470129472589,11.4));
#34359=CARTESIAN_POINT('Origin',(-3.05470129472589,3.05470129472589,11.4));
#34360=CARTESIAN_POINT('Origin',(-1.11809827484289,4.17279956956878,10.3684548175011));
#34361=CARTESIAN_POINT('',(-1.11809827484289,4.17279956956878,10.3369096350021));
#34362=CARTESIAN_POINT('',(-1.22309827484289,4.17279956956878,10.4));
#34363=CARTESIAN_POINT('',(-1.17059827484289,4.17279956956878,10.3684548175011));
#34364=CARTESIAN_POINT('Origin',(-1.11809827484289,4.17279956956878,10.4));
#34365=CARTESIAN_POINT('Origin',(-1.11809827484289,4.17279956956878,10.875));
#34366=CARTESIAN_POINT('',(-1.22309827484289,4.17279956956878,11.35));
#34367=CARTESIAN_POINT('',(-1.22309827484289,4.17279956956878,10.875));
#34368=CARTESIAN_POINT('Origin',(-1.11809827484289,4.17279956956878,11.35));
#34369=CARTESIAN_POINT('Origin',(-1.11809827484289,4.17279956956878,11.4));
#34370=CARTESIAN_POINT('',(-1.27309827484289,4.17279956956878,11.4));
#34371=CARTESIAN_POINT('',(-1.27309827484289,4.17279956956878,11.4));
#34372=CARTESIAN_POINT('Origin',(-1.11809827484289,4.17279956956878,11.4));
#34373=CARTESIAN_POINT('Origin',(1.11809827484289,4.17279956956878,10.3684548175011));
#34374=CARTESIAN_POINT('',(1.11809827484289,4.17279956956878,10.3369096350021));
#34375=CARTESIAN_POINT('',(1.01309827484289,4.17279956956878,10.4));
#34376=CARTESIAN_POINT('',(1.06559827484289,4.17279956956878,10.3684548175011));
#34377=CARTESIAN_POINT('Origin',(1.11809827484289,4.17279956956878,10.4));
#34378=CARTESIAN_POINT('Origin',(1.11809827484289,4.17279956956878,10.875));
#34379=CARTESIAN_POINT('',(1.01309827484289,4.17279956956878,11.35));
#34380=CARTESIAN_POINT('',(1.01309827484289,4.17279956956878,10.875));
#34381=CARTESIAN_POINT('Origin',(1.11809827484289,4.17279956956878,11.35));
#34382=CARTESIAN_POINT('Origin',(1.11809827484289,4.17279956956878,11.4));
#34383=CARTESIAN_POINT('',(0.96309827484289,4.17279956956878,11.4));
#34384=CARTESIAN_POINT('',(0.96309827484289,4.17279956956878,11.4));
#34385=CARTESIAN_POINT('Origin',(1.11809827484289,4.17279956956878,11.4));
#34386=CARTESIAN_POINT('Origin',(3.05470129472589,3.05470129472589,10.3684548175011));
#34387=CARTESIAN_POINT('',(3.05470129472589,3.05470129472589,10.3369096350021));
#34388=CARTESIAN_POINT('',(2.94970129472589,3.05470129472589,10.4));
#34389=CARTESIAN_POINT('',(3.00220129472589,3.05470129472589,10.3684548175011));
#34390=CARTESIAN_POINT('Origin',(3.05470129472589,3.05470129472589,10.4));
#34391=CARTESIAN_POINT('Origin',(3.05470129472589,3.05470129472589,10.875));
#34392=CARTESIAN_POINT('',(2.94970129472589,3.05470129472589,11.35));
#34393=CARTESIAN_POINT('',(2.94970129472589,3.05470129472589,10.875));
#34394=CARTESIAN_POINT('Origin',(3.05470129472589,3.05470129472589,11.35));
#34395=CARTESIAN_POINT('Origin',(3.05470129472589,3.05470129472589,11.4));
#34396=CARTESIAN_POINT('',(2.89970129472589,3.05470129472589,11.4));
#34397=CARTESIAN_POINT('',(2.89970129472589,3.05470129472589,11.4));
#34398=CARTESIAN_POINT('Origin',(3.05470129472589,3.05470129472589,11.4));
#34399=CARTESIAN_POINT('Origin',(4.17279956956878,1.11809827484289,10.3684548175011));
#34400=CARTESIAN_POINT('',(4.17279956956878,1.11809827484289,10.3369096350021));
#34401=CARTESIAN_POINT('',(4.06779956956878,1.11809827484289,10.4));
#34402=CARTESIAN_POINT('',(4.12029956956878,1.11809827484289,10.3684548175011));
#34403=CARTESIAN_POINT('Origin',(4.17279956956878,1.11809827484289,10.4));
#34404=CARTESIAN_POINT('Origin',(4.17279956956878,1.11809827484289,10.875));
#34405=CARTESIAN_POINT('',(4.06779956956878,1.11809827484289,11.35));
#34406=CARTESIAN_POINT('',(4.06779956956878,1.11809827484289,10.875));
#34407=CARTESIAN_POINT('Origin',(4.17279956956878,1.11809827484289,11.35));
#34408=CARTESIAN_POINT('Origin',(4.17279956956878,1.11809827484289,11.4));
#34409=CARTESIAN_POINT('',(4.01779956956878,1.11809827484289,11.4));
#34410=CARTESIAN_POINT('',(4.01779956956878,1.11809827484289,11.4));
#34411=CARTESIAN_POINT('Origin',(4.17279956956878,1.11809827484289,11.4));
#34412=CARTESIAN_POINT('Origin',(0.,0.,1.415));
#34413=CARTESIAN_POINT('',(4.13,-5.05779128047857E-16,1.4));
#34414=CARTESIAN_POINT('Origin',(0.,0.,1.4));
#34415=CARTESIAN_POINT('',(4.1,5.02105187650415E-16,1.43));
#34416=CARTESIAN_POINT('',(4.115,-5.03942157849136E-16,1.415));
#34417=CARTESIAN_POINT('',(-4.1,-5.02105187650415E-16,1.43));
#34418=CARTESIAN_POINT('Origin',(0.,0.,1.43));
#34419=CARTESIAN_POINT('Origin',(0.,0.,1.43));
#34420=CARTESIAN_POINT('Origin',(0.,0.,6.4));
#34421=CARTESIAN_POINT('',(4.1,-5.02105187650415E-16,11.37));
#34422=CARTESIAN_POINT('',(-4.1,-5.02105187650415E-16,11.37));
#34423=CARTESIAN_POINT('Origin',(0.,0.,11.37));
#34424=CARTESIAN_POINT('Origin',(0.,0.,11.37));
#34425=CARTESIAN_POINT('',(-4.1,-5.02105187650415E-16,6.4));
#34426=CARTESIAN_POINT('Origin',(4.6,0.,1.4));
#34427=CARTESIAN_POINT('',(4.56,5.58438940411193E-16,1.4));
#34428=CARTESIAN_POINT('Origin',(0.,0.,1.4));
#34429=CARTESIAN_POINT('Origin',(0.,0.,11.385));
#34430=CARTESIAN_POINT('',(4.13,5.05779128047857E-16,11.4));
#34431=CARTESIAN_POINT('',(4.115,-5.03942157849136E-16,11.385));
#34432=CARTESIAN_POINT('Origin',(0.,0.,11.4));
#34433=CARTESIAN_POINT('Origin',(4.1,0.,11.4));
#34434=CARTESIAN_POINT('',(4.56,-5.58438940411193E-16,11.4));
#34435=CARTESIAN_POINT('Origin',(0.,0.,11.4));
#34436=CARTESIAN_POINT('Origin',(0.,0.,11.38));
#34437=CARTESIAN_POINT('',(4.6,5.63337527607782E-16,11.36));
#34438=CARTESIAN_POINT('',(4.58,5.60888234009488E-16,11.38));
#34439=CARTESIAN_POINT('',(-4.6,-5.63337527607782E-16,11.36));
#34440=CARTESIAN_POINT('Origin',(0.,0.,11.36));
#34441=CARTESIAN_POINT('Origin',(0.,0.,11.36));
#34442=CARTESIAN_POINT('Origin',(0.,0.,6.4));
#34443=CARTESIAN_POINT('',(-4.6,-5.63337527607782E-16,1.44));
#34444=CARTESIAN_POINT('',(-4.6,-5.63337527607782E-16,6.4));
#34445=CARTESIAN_POINT('',(4.6,-5.63337527607782E-16,1.44));
#34446=CARTESIAN_POINT('Origin',(0.,0.,1.44));
#34447=CARTESIAN_POINT('Origin',(0.,0.,1.44));
#34448=CARTESIAN_POINT('Origin',(0.,0.,1.42));
#34449=CARTESIAN_POINT('',(4.58,5.60888234009488E-16,1.42));
#54961=UNCERTAINTY_MEASURE_WITH_UNIT(LENGTH_MEASURE(0.001),#55003,
'DISTANCE_ACCURACY_VALUE',
'Maximum model space distance between geometric entities at asserted c
onnectivities');
#54980=UNCERTAINTY_MEASURE_WITH_UNIT(LENGTH_MEASURE(0.001),#55003,
'DISTANCE_ACCURACY_VALUE',
'Maximum model space distance between geometric entities at asserted c
onnectivities');
#54983=(
GEOMETRIC_REPRESENTATION_CONTEXT(3)
GLOBAL_UNCERTAINTY_ASSIGNED_CONTEXT((#54961))
GLOBAL_UNIT_ASSIGNED_CONTEXT((#55003,#55005,#55006))
REPRESENTATION_CONTEXT('','3D')
);
#55002=(
GEOMETRIC_REPRESENTATION_CONTEXT(3)
GLOBAL_UNCERTAINTY_ASSIGNED_CONTEXT((#54980))
GLOBAL_UNIT_ASSIGNED_CONTEXT((#55003,#55005,#55006))
REPRESENTATION_CONTEXT('','3D')
);
#55003=(
LENGTH_UNIT()
NAMED_UNIT(*)
SI_UNIT(.CENTI.,.METRE.)
);
#55005=(
NAMED_UNIT(*)
PLANE_ANGLE_UNIT()
SI_UNIT($,.RADIAN.)
);
#55006=(
NAMED_UNIT(*)
SI_UNIT($,.STERADIAN.)
SOLID_ANGLE_UNIT()
);
#55009=SHAPE_DEFINITION_REPRESENTATION(#55030,#55105);
#55030=PRODUCT_DEFINITION_SHAPE('',$,#55127);
#55105=SHAPE_REPRESENTATION('',(#24929),#54983);
#55124=PRODUCT_DEFINITION_CONTEXT('part definition',#55189,'design');
#55127=PRODUCT_DEFINITION('2026-10-18-23-35-49-944',
'02_Chopper_Enclosure_Guard_Shield_D92',#55148,#55124);
#55148=PRODUCT_DEFINITION_FORMATION('',$,#55193);
#55189=APPLICATION_CONTEXT(
'Core Data for Automotive Mechanical Design Process');
#55190=PRODUCT_CONTEXT('part definition',#55189,'mechanical');
#55193=PRODUCT('2026-10-18-23-35-49-944',
'02_Chopper_Enclosure_Guard_Shield_D92',$,(#55190));
#55373=COLOUR_RGB('Sky Blue',0.24,0.69,0.87);
#55374=FILL_AREA_STYLE_COLOUR('',#55373);
#55375=FILL_AREA_STYLE('',(#55374));
#55376=SURFACE_STYLE_FILL_AREA(#55375);
#55377=SURFACE_SIDE_STYLE('',(#55376));
#55378=SURFACE_STYLE_USAGE(.BOTH.,#55377);
#55379=PRESENTATION_STYLE_ASSIGNMENT((#55378));
ENDSEC;
END-ISO-10303-21;
